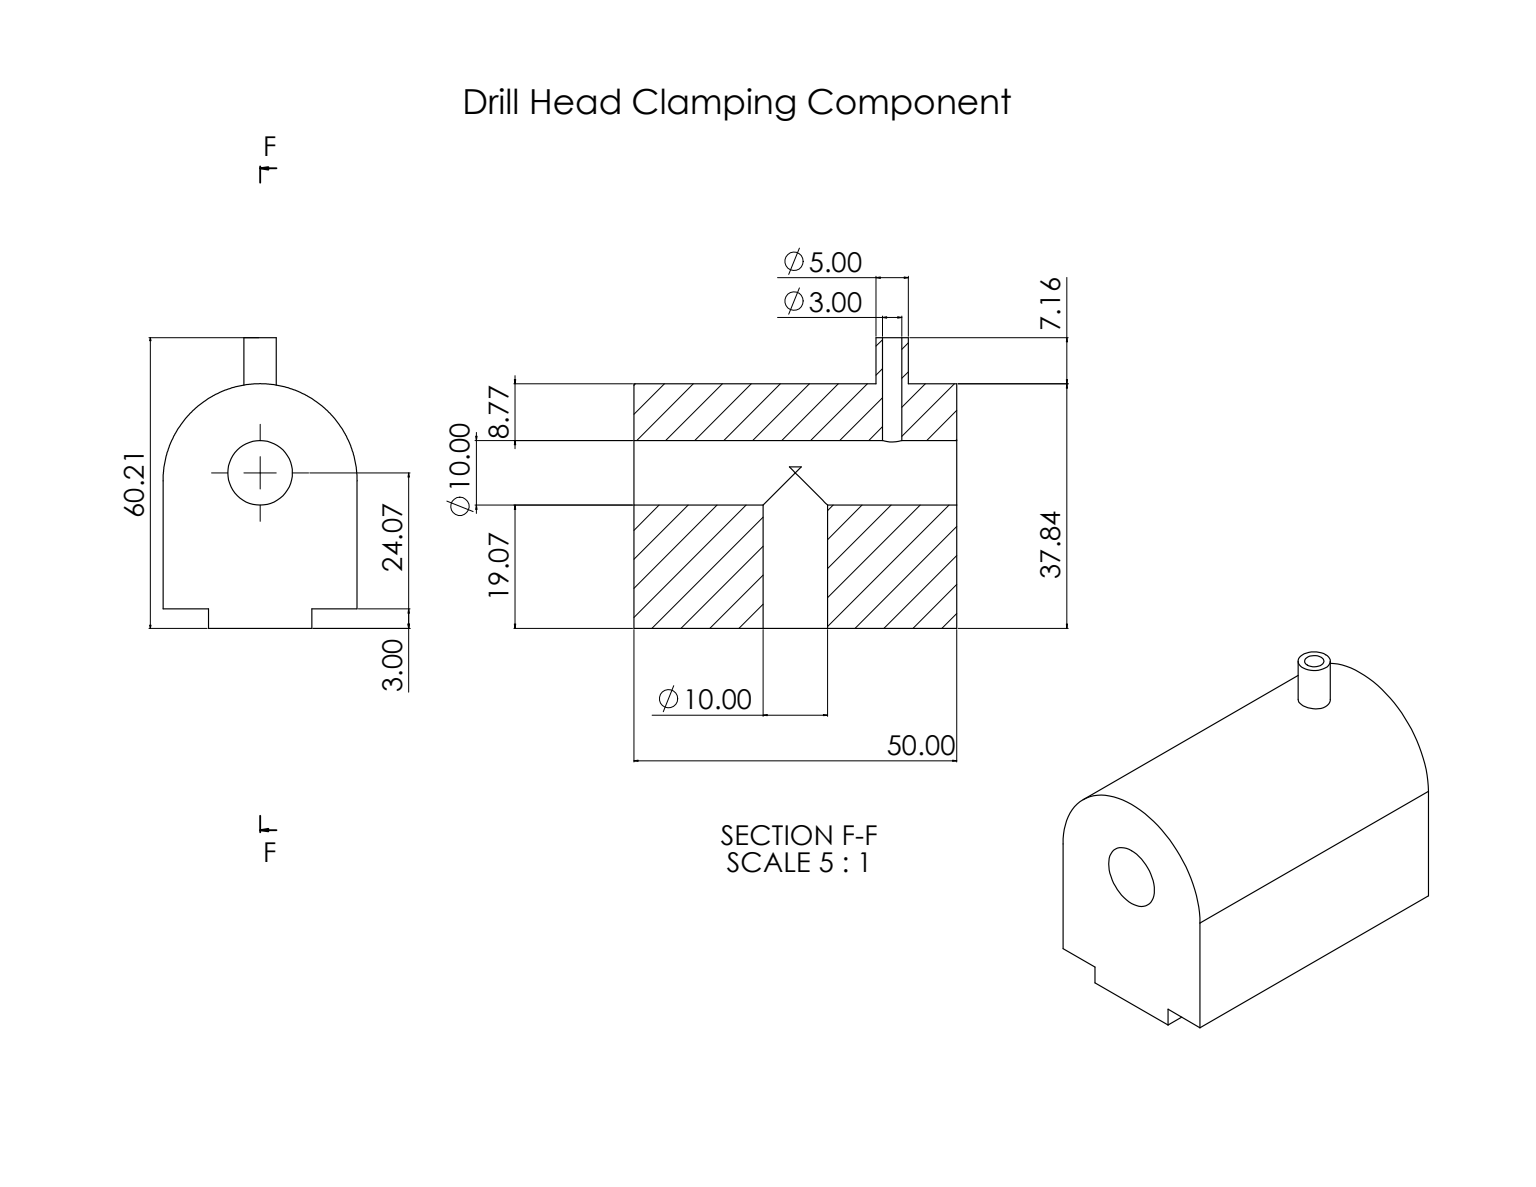
ISO-10303-21;
HEADER;
FILE_DESCRIPTION (('STEP AP214'),
    '1' );
FILE_NAME ('Drill Head Clamping Component.step',
    '2026-10-26T22:46:44',
    ( '' ),
    ( '' ),
    'SwSTEP 2.0',
    'SolidWorks 2025',
    '' );
FILE_SCHEMA (( 'AUTOMOTIVE_DESIGN' ));
ENDSEC;

DATA;
#26=DIRECTION ( 'NONE',  ( 0.5000000000000044409, -0.8660254037844360431, -4.006172263299080068E-16 ) ) ;
#120=CARTESIAN_POINT ( 'NONE',  ( 184.9952905943350743, 3.535126980567765642, 0.9999999999999187317 ) ) ;
#154=CARTESIAN_POINT ( 'NONE',  ( 189.6713070174558311, 31.72030020615783030, -9.000000000000065725 ) ) ;
#219=CARTESIAN_POINT ( 'NONE',  ( 203.2433706042751282, 14.07066088650062241, -14.00000000000004974 ) ) ;
#263=EDGE_CURVE ( 'NONE', #15664, #11736, #7688, .T. ) ;
#270=VERTEX_POINT ( 'NONE', #17044 ) ;
#297=AXIS2_PLACEMENT_3D ( 'NONE', #15625, #6046, #20370 ) ;
#298=CARTESIAN_POINT ( 'NONE',  ( 191.0833833835251880, 36.99024094849657018, -18.91295074164679235 ) ) ;
#299=( BOUNDED_CURVE ( )  B_SPLINE_CURVE ( 3, ( #3480, #412, #16318, #298 ),
 .UNSPECIFIED., .F., .F. ) 
 B_SPLINE_CURVE_WITH_KNOTS ( ( 4, 4 ),
 ( 1.570796326794896114, 1.757668500643543075 ),
 .UNSPECIFIED. ) 
 CURVE ( )  GEOMETRIC_REPRESENTATION_ITEM ( )  RATIONAL_B_SPLINE_CURVE ( ( 1.000000000000000000, 0.9970920157757051649, 0.9970920157757051649, 1.000000000000000000 ) ) 
 REPRESENTATION_ITEM ( '' )  );
#319=EDGE_CURVE ( 'NONE', #17948, #11709, #17482, .T. ) ;
#339=CARTESIAN_POINT ( 'NONE',  ( 203.2094460813901833, 24.04198982742622448, -13.33402418452071814 ) ) ;
#363=VECTOR ( 'NONE', #26, 1000.000000000000114 ) ;
#394=ORIENTED_EDGE ( 'NONE', *, *, #20392, .T. ) ;
#410=ORIENTED_EDGE ( 'NONE', *, *, #16561, .T. ) ;
#412=CARTESIAN_POINT ( 'NONE',  ( 190.8575367324608294, 36.14736977200441004, -19.00000000000003908 ) ) ;
#450=CARTESIAN_POINT ( 'NONE',  ( 201.8234976231972553, 26.52995303002162331, -14.00000000000004619 ) ) ;
#462=LINE ( 'NONE', #18261, #4286 ) ;
#465=ORIENTED_EDGE ( 'NONE', *, *, #17085, .T. ) ;
#502=ORIENTED_EDGE ( 'NONE', *, *, #9754, .F. ) ;
#521=CARTESIAN_POINT ( 'NONE',  ( 190.7433706042750146, 35.72129598111152404, -19.00000000000003908 ) ) ;
#586=CARTESIAN_POINT ( 'NONE',  ( 191.5478494775925640, 36.18576207517880050, -14.00000000000006395 ) ) ;
#601=ORIENTED_EDGE ( 'NONE', *, *, #10960, .T. ) ;
#656=ORIENTED_EDGE ( 'NONE', *, *, #14023, .F. ) ;
#665=EDGE_CURVE ( 'NONE', #15359, #17948, #14273, .T. ) ;
#674=FACE_OUTER_BOUND ( 'NONE', #15043, .T. ) ;
#709=VECTOR ( 'NONE', #16147, 1000.000000000000000 ) ;
#716=DIRECTION ( 'NONE',  ( 0.5000000000000046629, -0.8660254037844360431, -4.006172263299081054E-16 ) ) ;
#719=ADVANCED_FACE ( 'NONE', ( #9867 ), #20902, .F. ) ;
#723=EDGE_CURVE ( 'NONE', #3430, #270, #9321, .T. ) ;
#750=LINE ( 'NONE', #16854, #10405 ) ;
#778=ORIENTED_EDGE ( 'NONE', *, *, #1234, .T. ) ;
#783=PRODUCT ( 'Drill Head Clamping Component', 'Drill Head Clamping Component', '', ( #7533 ) ) ;
#784=VERTEX_POINT ( 'NONE', #1941 ) ;
#837=CARTESIAN_POINT ( 'NONE',  ( 201.9048419744482317, 26.22127161638350756, -13.08418984338544355 ) ) ;
#849=LINE ( 'NONE', #4134, #8722 ) ;
#861=EDGE_CURVE ( 'NONE', #17088, #19623, #11689, .T. ) ;
#939=CARTESIAN_POINT ( 'NONE',  ( 201.8234976231972269, 26.52995303002161620, -13.90027237864162757 ) ) ;
#942=VECTOR ( 'NONE', #9777, 1000.000000000000114 ) ;
#946=ORIENTED_EDGE ( 'NONE', *, *, #6874, .T. ) ;
#962=EDGE_CURVE ( 'NONE', #14228, #10601, #3174, .T. ) ;
#978=ORIENTED_EDGE ( 'NONE', *, *, #6131, .F. ) ;
#1019=DIRECTION ( 'NONE',  ( -3.517351572405780687E-16, 2.595185392108431646E-16, -1.000000000000000000 ) ) ;
#1071=DIRECTION ( 'NONE',  ( -0.8660254037844361541, -0.5000000000000045519, -4.336808689942050770E-16 ) ) ;
#1074=PLANE ( 'NONE',  #8585 ) ;
#1129=EDGE_CURVE ( 'NONE', #19322, #784, #1828, .T. ) ;
#1234=EDGE_CURVE ( 'NONE', #10655, #15958, #18417, .T. ) ;
#1236=ORIENTED_EDGE ( 'NONE', *, *, #11597, .T. ) ;
#1267=EDGE_CURVE ( 'NONE', #13023, #3226, #5866, .T. ) ;
#1274=DIRECTION ( 'NONE',  ( 0.000000000000000000, 0.000000000000000000, 1.000000000000000000 ) ) ;
#1300=CARTESIAN_POINT ( 'NONE',  ( 210.6607590550263183, 28.44678604684768786, -16.18447207777755281 ) ) ;
#1305=DIRECTION ( 'NONE',  ( 0.5000000000000044409, -0.8660254037844360431, 0.000000000000000000 ) ) ;
#1311=DIRECTION ( 'NONE',  ( 0.5000000000000046629, -0.8660254037844360431, -4.006172263299081054E-16 ) ) ;
#1339=CARTESIAN_POINT ( 'NONE',  ( 203.3234976231972553, 23.93187681866832861, -14.00000000000004441 ) ) ;
#1341=DIRECTION ( 'NONE',  ( 0.8660254037844360431, 0.5000000000000044409, 4.336808689942049290E-16 ) ) ;
#1403=CARTESIAN_POINT ( 'NONE',  ( 215.1694833127197057, 20.95620526910698445, -14.00000000000008527 ) ) ;
#1430=VECTOR ( 'NONE', #5416, 1000.000000000000227 ) ;
#1434=CARTESIAN_POINT ( 'NONE',  ( 188.9132435853528591, 28.89116896218934016, -16.92893218813457068 ) ) ;
#1459=DIRECTION ( 'NONE',  ( 0.5000000000000044409, -0.8660254037844360431, -4.006172263299080068E-16 ) ) ;
#1464=DIRECTION ( 'NONE',  ( 0.5000000000000057732, -0.8660254037844353769, 0.000000000000000000 ) ) ;
#1500=DIRECTION ( 'NONE',  ( -0.5000000000000025535, 0.8660254037844372643, 0.000000000000000000 ) ) ;
#1504=CARTESIAN_POINT ( 'NONE',  ( 210.0699630922315748, 29.36925333534437499, -16.49993777872327527 ) ) ;
#1510=PLANE ( 'NONE',  #13226 ) ;
#1512=DIRECTION ( 'NONE',  ( -0.8660254037844361541, -0.5000000000000045519, 8.850264995343375625E-15 ) ) ;
#1579=CIRCLE ( 'NONE', #13424, 15.00000000000001954 ) ;
#1607=CARTESIAN_POINT ( 'NONE',  ( 209.1488401613018198, 31.20282942076142518, -15.65137675853565646 ) ) ;
#1621=DIRECTION ( 'NONE',  ( 0.8660254037844361541, 0.5000000000000044409, 0.000000000000000000 ) ) ;
#1642=CARTESIAN_POINT ( 'NONE',  ( 188.9132435853528591, 28.89116896218934016, -11.07106781186553768 ) ) ;
#1649=CARTESIAN_POINT ( 'NONE',  ( 210.8166463470705310, 28.23117696587115333, -12.01093917984183790 ) ) ;
#1691=CARTESIAN_POINT ( 'NONE',  ( 184.9952905943350743, 3.535126980567779409, -29.00000000000008882 ) ) ;
#1702=ORIENTED_EDGE ( 'NONE', *, *, #12220, .F. ) ;
#1749=ADVANCED_FACE ( 'NONE', ( #8633 ), #15030, .F. ) ;
#1752=CARTESIAN_POINT ( 'NONE',  ( 211.3365836822136430, 27.55273924158569798, -13.19013634410915969 ) ) ;
#1828=CIRCLE ( 'NONE', #18066, 1.499999999999993783 ) ;
#1869=( NAMED_UNIT ( * ) PLANE_ANGLE_UNIT ( ) SI_UNIT ( $, .RADIAN. ) );
#1875=AXIS2_PLACEMENT_3D ( 'NONE', #4980, #8260, #18132 ) ;
#1896=ADVANCED_FACE ( 'NONE', ( #19128 ), #2497, .F. ) ;
#1902=DIRECTION ( 'NONE',  ( -2.003086131649568876E-16, 3.469446951953589044E-16, -1.000000000000000000 ) ) ;
#1934=CARTESIAN_POINT ( 'NONE',  ( 201.8352585209308359, 26.48094985263767498, -13.60979871437957911 ) ) ;
#1941=CARTESIAN_POINT ( 'NONE',  ( 217.1183575532814416, 31.89634291273570810, -14.00000000000004441 ) ) ;
#1972=CARTESIAN_POINT ( 'NONE',  ( 203.2093925786781767, 24.04204282662517400, -14.66612357830583946 ) ) ;
#1979=EDGE_LOOP ( 'NONE', ( #13601, #10740, #15513, #394 ) ) ;
#1980=ORIENTED_EDGE ( 'NONE', *, *, #665, .T. ) ;
#1988=ORIENTED_EDGE ( 'NONE', *, *, #20436, .F. ) ;
#1996=ORIENTED_EDGE ( 'NONE', *, *, #12220, .T. ) ;
#2021=ORIENTED_EDGE ( 'NONE', *, *, #14700, .T. ) ;
#2053=LINE ( 'NONE', #5528, #1430 ) ;
#2091=EDGE_LOOP ( 'NONE', ( #13331, #5335, #14741, #12606, #6343, #16377, #14233, #11644, #18125 ) ) ;
#2162=CARTESIAN_POINT ( 'NONE',  ( 202.1791022559531541, 13.45620526910691694, -14.00000000000008527 ) ) ;
#2272=EDGE_LOOP ( 'NONE', ( #3905, #20020, #978 ) ) ;
#2294=DIRECTION ( 'NONE',  ( -0.5000000000000034417, 0.8660254037844364872, 0.000000000000000000 ) ) ;
#2335=ORIENTED_EDGE ( 'NONE', *, *, #4367, .F. ) ;
#2396=DIRECTION ( 'NONE',  ( -0.8660254037844360431, -0.5000000000000045519, -4.336808689942049784E-16 ) ) ;
#2409=CARTESIAN_POINT ( 'NONE',  ( 173.9132435853527454, 54.87193107572242212, -14.00000000000002842 ) ) ;
#2410=CIRCLE ( 'NONE', #14943, 4.999999999999978684 ) ;
#2415=ORIENTED_EDGE ( 'NONE', *, *, #11750, .F. ) ;
#2433=ORIENTED_EDGE ( 'NONE', *, *, #20050, .T. ) ;
#2462=ORIENTED_EDGE ( 'NONE', *, *, #1234, .F. ) ;
#2476=( BOUNDED_CURVE ( )  B_SPLINE_CURVE ( 3, ( #8745, #4299, #15659, #5761 ),
 .UNSPECIFIED., .F., .F. ) 
 B_SPLINE_CURVE_WITH_KNOTS ( ( 4, 4 ),
 ( 1.383924152946250041, 1.570796326794896558 ),
 .UNSPECIFIED. ) 
 CURVE ( )  GEOMETRIC_REPRESENTATION_ITEM ( )  RATIONAL_B_SPLINE_CURVE ( ( 1.000000000000000000, 0.9970920157757051649, 0.9970920157757051649, 1.000000000000000000 ) ) 
 REPRESENTATION_ITEM ( '' )  );
#2482=ORIENTED_EDGE ( 'NONE', *, *, #20787, .T. ) ;
#2485=LINE ( 'NONE', #7338, #20363 ) ;
#2497=CYLINDRICAL_SURFACE ( 'NONE', #8268, 4.999999999999975131 ) ;
#2514=CARTESIAN_POINT ( 'NONE',  ( 177.1791022559528983, 56.75747545832873442, -29.00000000000007105 ) ) ;
#2536=CARTESIAN_POINT ( 'NONE',  ( 201.8258408404966531, 26.51993709131365762, -13.80232238285611857 ) ) ;
#2568=CIRCLE ( 'NONE', #1875, 15.00000000000001954 ) ;
#2571=AXIS2_PLACEMENT_3D ( 'NONE', #13843, #5653, #14253 ) ;
#2577=EDGE_LOOP ( 'NONE', ( #4212, #6761 ) ) ;
#2578=CARTESIAN_POINT ( 'NONE',  ( 203.2433706042751282, 14.07066088650062241, -14.00000000000004974 ) ) ;
#2611=ORIENTED_EDGE ( 'NONE', *, *, #17969, .F. ) ;
#2632=CARTESIAN_POINT ( 'NONE',  ( 216.3683575532813848, 33.19538101841231992, -14.00000000000004441 ) ) ;
#2635=CARTESIAN_POINT ( 'NONE',  ( 207.5734976231972837, 16.57066088650062241, -14.00000000000004974 ) ) ;
#2657=PRODUCT_DEFINITION_SHAPE ( 'NONE', 'NONE',  #13142 ) ;
#2676=( GEOMETRIC_REPRESENTATION_CONTEXT ( 3 ) GLOBAL_UNCERTAINTY_ASSIGNED_CONTEXT ( ( #17640 ) ) GLOBAL_UNIT_ASSIGNED_CONTEXT ( ( #13415, #7036, #20186 ) ) REPRESENTATION_CONTEXT ( 'NONE', 'WORKASPACE' ) );
#2716=FACE_OUTER_BOUND ( 'NONE', #2577, .T. ) ;
#2720=VERTEX_POINT ( 'NONE', #6853 ) ;
#2721=ORIENTED_EDGE ( 'NONE', *, *, #14023, .T. ) ;
#2733=DIRECTION ( 'NONE',  ( 0.5000000000000015543, -0.8660254037844377084, 0.000000000000000000 ) ) ;
#2811=VECTOR ( 'NONE', #20786, 1000.000000000000114 ) ;
#2817=LINE ( 'NONE', #17224, #20375 ) ;
#2860=VERTEX_POINT ( 'NONE', #10871 ) ;
#2888=CARTESIAN_POINT ( 'NONE',  ( 209.4688803963327928, 30.49173192974595992, -16.24689738482229728 ) ) ;
#2890=EDGE_LOOP ( 'NONE', ( #656, #6702, #11561, #1980, #5146 ) ) ;
#2893=DIRECTION ( 'NONE',  ( 0.5000000000000044409, -0.8660254037844360431, 0.000000000000000000 ) ) ;
#2924=VECTOR ( 'NONE', #8682, 1000.000000000000114 ) ;
#2937=ORIENTED_EDGE ( 'NONE', *, *, #263, .T. ) ;
#3047=DIRECTION ( 'NONE',  ( 0.5000000000000046629, -0.8660254037844360431, -4.006172263299081054E-16 ) ) ;
#3097=CARTESIAN_POINT ( 'NONE',  ( 208.9194833127196489, 31.78152281641241572, -14.16331216883973987 ) ) ;
#3104=CARTESIAN_POINT ( 'NONE',  ( 190.7433706042750146, 35.72129598111152404, -9.000000000000062172 ) ) ;
#3137=CARTESIAN_POINT ( 'NONE',  ( 209.4677058171011197, 30.49417139021348078, -11.75443427544081310 ) ) ;
#3174=CIRCLE ( 'NONE', #10608, 5.000000000000002665 ) ;
#3193=CARTESIAN_POINT ( 'NONE',  ( 210.4099586451761184, 28.82287685411301936, -16.37159109994057360 ) ) ;
#3219=VECTOR ( 'NONE', #13608, 1000.000000000000114 ) ;
#3226=VERTEX_POINT ( 'NONE', #18596 ) ;
#3251=DIRECTION ( 'NONE',  ( -0.8660254037844360431, -0.5000000000000045519, -4.336808689942050277E-16 ) ) ;
#3295=CARTESIAN_POINT ( 'NONE',  ( 209.8259871216629335, 29.79736469536937093, -16.48372795108025812 ) ) ;
#3338=CARTESIAN_POINT ( 'NONE',  ( 209.6745996013020772, 30.08081452043873227, -11.58037181831264029 ) ) ;
#3358=B_SPLINE_CURVE_WITH_KNOTS ( 'NONE', 3,
 ( #14921, #7255, #8744, #1972, #15242, #19978, #13638, #20091, #16912, #15037, #8536, #12042, #18607, #18289, #13738, #10320, #15139, #11829, #16595, #8639, #5441, #3763, #11940, #18509, #5235, #5552, #13425, #15350 ),
 .UNSPECIFIED., .F., .F.,
 ( 4, 2, 2, 2, 2, 2, 2, 2, 2, 2, 2, 2, 2, 4 ),
 ( 0.004717002832140601738, 0.005306469451344702354, 0.005601202760946753095, 0.005895936070548802969, 0.006485402689752946953, 0.006780135999355018511, 0.007074869308957089202, 0.007369602618559159893, 0.007664335928161231451, 0.008253802547365364159, 0.008548535856967442656, 0.008843269166569519418, 0.009138002476171597915, 0.009432735785773674678 ),
 .UNSPECIFIED. ) ;
#3368=AXIS2_PLACEMENT_3D ( 'NONE', #10550, #17528, #1621 ) ;
#3392=CIRCLE ( 'NONE', #13898, 2.499999999999994671 ) ;
#3430=VERTEX_POINT ( 'NONE', #15661 ) ;
#3480=CARTESIAN_POINT ( 'NONE',  ( 190.7433706042750146, 35.72129598111152404, -19.00000000000003908 ) ) ;
#3710=DIRECTION ( 'NONE',  ( 0.5000000000000044409, -0.8660254037844360431, -4.006172263299080068E-16 ) ) ;
#3734=CARTESIAN_POINT ( 'NONE',  ( 159.9952905943348469, 46.83639716978957068, 0.9999999999999386047 ) ) ;
#3754=SHAPE_REPRESENTATION_RELATIONSHIP ( 'NONE' , 'NONE' ,  #9638, #5517 ) ;
#3756=VERTEX_POINT ( 'NONE', #15220 ) ;
#3762=ORIENTED_EDGE ( 'NONE', *, *, #16561, .F. ) ;
#3763=CARTESIAN_POINT ( 'NONE',  ( 201.8742535751798073, 26.32928792145338548, -14.75325243452065749 ) ) ;
#3767=DIRECTION ( 'NONE',  ( 0.8660254037844360431, 0.5000000000000045519, 4.336808689942049784E-16 ) ) ;
#3773=ORIENTED_EDGE ( 'NONE', *, *, #14700, .F. ) ;
#3778=ORIENTED_EDGE ( 'NONE', *, *, #319, .F. ) ;
#3805=ORIENTED_EDGE ( 'NONE', *, *, #13350, .T. ) ;
#3828=DIRECTION ( 'NONE',  ( 0.8660254037844360431, 0.5000000000000045519, 4.336808689942050277E-16 ) ) ;
#3905=ORIENTED_EDGE ( 'NONE', *, *, #8879, .F. ) ;
#3927=LINE ( 'NONE', #8806, #11231 ) ;
#3983=DIRECTION ( 'NONE',  ( -0.8660254037844360431, -0.5000000000000044409, -4.336808689942049290E-16 ) ) ;
#4002=LINE ( 'NONE', #18212, #14326 ) ;
#4009=CARTESIAN_POINT ( 'NONE',  ( 202.1874421558074744, 25.46507160306319406, -12.54005369788149693 ) ) ;
#4012=VERTEX_POINT ( 'NONE', #18044 ) ;
#4100=AXIS2_PLACEMENT_3D ( 'NONE', #17999, #3251, #1464 ) ;
#4134=CARTESIAN_POINT ( 'NONE',  ( 159.9952905943348469, 46.83639716978957068, 0.9999999999999386047 ) ) ;
#4180=FACE_OUTER_BOUND ( 'NONE', #1979, .T. ) ;
#4198=ADVANCED_FACE ( 'NONE', ( #5801, #12295 ), #7500, .T. ) ;
#4207=( BOUNDED_CURVE ( )  B_SPLINE_CURVE ( 3, ( #16447, #11575, #14992, #18045 ),
 .UNSPECIFIED., .F., .F. ) 
 B_SPLINE_CURVE_WITH_KNOTS ( ( 4, 4 ),
 ( 4.525516806536070469, 4.712388980384689674 ),
 .UNSPECIFIED. ) 
 CURVE ( )  GEOMETRIC_REPRESENTATION_ITEM ( )  RATIONAL_B_SPLINE_CURVE ( ( 1.000000000000000000, 0.9970920157757060531, 0.9970920157757060531, 1.000000000000000000 ) ) 
 REPRESENTATION_ITEM ( '' )  );
#4212=ORIENTED_EDGE ( 'NONE', *, *, #10396, .T. ) ;
#4227=VERTEX_POINT ( 'NONE', #7385 ) ;
#4286=VECTOR ( 'NONE', #18474, 1000.000000000000114 ) ;
#4299=CARTESIAN_POINT ( 'NONE',  ( 191.5936596622673278, 35.49346171468947375, -18.97089895516968028 ) ) ;
#4323=CARTESIAN_POINT ( 'NONE',  ( 191.0833833835251880, 36.99024094849657018, -18.91295074164679235 ) ) ;
#4340=EDGE_LOOP ( 'NONE', ( #11227, #4467, #18364, #14808, #8937, #2021, #8246, #17322, #3805 ) ) ;
#4367=EDGE_CURVE ( 'NONE', #11709, #17948, #17634, .T. ) ;
#4383=CARTESIAN_POINT ( 'NONE',  ( 159.9952905943347901, 46.83639716978955647, -22.00000000000007816 ) ) ;
#4388=DIRECTION ( 'NONE',  ( 1.561274065702232331E-18, -4.616915249250367527E-16, 1.000000000000000000 ) ) ;
#4461=DIRECTION ( 'NONE',  ( -0.5000000000000045519, 0.8660254037844360431, 4.006172263299081054E-16 ) ) ;
#4467=ORIENTED_EDGE ( 'NONE', *, *, #16106, .T. ) ;
#4485=LINE ( 'NONE', #12339, #5183 ) ;
#4486=FACE_OUTER_BOUND ( 'NONE', #4840, .T. ) ;
#4584=CARTESIAN_POINT ( 'NONE',  ( 217.6183575532813848, 31.03031750895123508, -14.00000000000004441 ) ) ;
#4598=CARTESIAN_POINT ( 'NONE',  ( 191.5478494775925640, 36.18576207517880050, -14.00000000000006395 ) ) ;
#4622=EDGE_CURVE ( 'NONE', #9607, #13077, #8793, .T. ) ;
#4652=DIRECTION ( 'NONE',  ( -0.8660254037844344888, -0.5000000000000069944, 0.000000000000000000 ) ) ;
#4715=EDGE_CURVE ( 'NONE', #18333, #14531, #8447, .T. ) ;
#4717=CARTESIAN_POINT ( 'NONE',  ( 209.1489059746362216, 31.20269758479947697, -12.34862215763092763 ) ) ;
#4731=ADVANCED_FACE ( 'NONE', ( #11058 ), #7759, .T. ) ;
#4777=CARTESIAN_POINT ( 'NONE',  ( 216.3683575532814416, 33.19538101841234834, -14.00000000000004441 ) ) ;
#4831=VECTOR ( 'NONE', #15686, 1000.000000000000114 ) ;
#4840=EDGE_LOOP ( 'NONE', ( #9568, #10904, #6846, #9175 ) ) ;
#4867=ORIENTED_EDGE ( 'NONE', *, *, #7845, .T. ) ;
#4884=ORIENTED_EDGE ( 'NONE', *, *, #6131, .T. ) ;
#4886=CARTESIAN_POINT ( 'NONE',  ( 210.1535261002520087, 29.22995462719417148, -16.48401562083277483 ) ) ;
#4894=EDGE_LOOP ( 'NONE', ( #11762, #6045, #20022 ) ) ;
#4922=CARTESIAN_POINT ( 'NONE',  ( 159.9952905943347901, 46.83639716978955647, -22.00000000000007816 ) ) ;
#4957=CARTESIAN_POINT ( 'NONE',  ( 157.3972143829815309, 45.33639716978957068, -22.00000000000007816 ) ) ;
#4973=ORIENTED_EDGE ( 'NONE', *, *, #6796, .F. ) ;
#4980=CARTESIAN_POINT ( 'NONE',  ( 177.1791022559528983, 56.75747545832872731, -14.00000000000006395 ) ) ;
#5014=EDGE_CURVE ( 'NONE', #784, #19322, #12224, .T. ) ;
#5022=DIRECTION ( 'NONE',  ( -0.8660254037844361541, -0.5000000000000045519, -8.850264995343378780E-15 ) ) ;
#5033=( NAMED_UNIT ( * ) SI_UNIT ( $, .STERADIAN. ) SOLID_ANGLE_UNIT ( ) );
#5076=DIRECTION ( 'NONE',  ( 0.5000000000000046629, -0.8660254037844360431, -4.006172263299081054E-16 ) ) ;
#5083=CARTESIAN_POINT ( 'NONE',  ( 191.5478494775925640, 36.18576207517880050, -14.00000000000006395 ) ) ;
#5118=CARTESIAN_POINT ( 'NONE',  ( 188.9132435853528591, 28.89116896218935082, -14.00000000000004086 ) ) ;
#5138=CARTESIAN_POINT ( 'NONE',  ( 159.9952905943347901, 46.83639716978954226, -6.000000000000052403 ) ) ;
#5146=ORIENTED_EDGE ( 'NONE', *, *, #319, .T. ) ;
#5170=ORIENTED_EDGE ( 'NONE', *, *, #7845, .F. ) ;
#5183=VECTOR ( 'NONE', #14256, 1000.000000000000114 ) ;
#5193=CARTESIAN_POINT ( 'NONE',  ( 202.2752485137783083, 25.28694651298519958, -12.50009056643368943 ) ) ;
#5235=CARTESIAN_POINT ( 'NONE',  ( 201.8352900073124658, 26.48082042610822029, -14.39073202032135335 ) ) ;
#5240=CARTESIAN_POINT ( 'NONE',  ( 216.3683575532813848, 33.19538101841231992, -14.00000000000004441 ) ) ;
#5284=CARTESIAN_POINT ( 'NONE',  ( 184.9952905943350459, 3.535126980567751431, -22.00000000000009948 ) ) ;
#5285=AXIS2_PLACEMENT_3D ( 'NONE', #4922, #5022, #11398 ) ;
#5294=CARTESIAN_POINT ( 'NONE',  ( 201.9876756982950781, 25.95812089196162020, -12.80147382135962353 ) ) ;
#5295=EDGE_CURVE ( 'NONE', #17359, #17685, #10465, .T. ) ;
#5335=ORIENTED_EDGE ( 'NONE', *, *, #15580, .F. ) ;
#5341=DIRECTION ( 'NONE',  ( 0.5000000000000015543, -0.8660254037844377084, 0.000000000000000000 ) ) ;
#5395=AXIS2_PLACEMENT_3D ( 'NONE', #16816, #3767, #2294 ) ;
#5416=DIRECTION ( 'NONE',  ( 0.8660254037844344888, 0.5000000000000069944, 0.000000000000000000 ) ) ;
#5426=ORIENTED_EDGE ( 'NONE', *, *, #14613, .F. ) ;
#5441=CARTESIAN_POINT ( 'NONE',  ( 201.9048576179487213, 26.22121821873378877, -14.91588034066295521 ) ) ;
#5443=FACE_BOUND ( 'NONE', #20780, .T. ) ;
#5462=AXIS2_PLACEMENT_3D ( 'NONE', #2162, #8615, #7123 ) ;
#5517=ADVANCED_BREP_SHAPE_REPRESENTATION ( '', ( #10635, #18233 ), #2676 ) ;
#5528=CARTESIAN_POINT ( 'NONE',  ( 182.3972143829817867, 2.035126980567763866, -22.00000000000009948 ) ) ;
#5552=CARTESIAN_POINT ( 'NONE',  ( 201.8258405466010572, 26.51993739047028242, -14.19778417152125805 ) ) ;
#5569=ORIENTED_EDGE ( 'NONE', *, *, #17776, .T. ) ;
#5653=DIRECTION ( 'NONE',  ( 0.8660254037844360431, 0.5000000000000045519, 4.336808689942049784E-16 ) ) ;
#5708=CARTESIAN_POINT ( 'NONE',  ( 177.1791022559528983, 56.75747545832872731, -29.00000000000007105 ) ) ;
#5715=DIRECTION ( 'NONE',  ( -0.5000000000000025535, 0.8660254037844372643, 0.000000000000000000 ) ) ;
#5761=CARTESIAN_POINT ( 'NONE',  ( 190.7433706042750146, 35.72129598111152404, -19.00000000000003908 ) ) ;
#5781=DIRECTION ( 'NONE',  ( -0.8660254037844361541, -0.5000000000000044409, 0.000000000000000000 ) ) ;
#5798=ORIENTED_EDGE ( 'NONE', *, *, #6374, .F. ) ;
#5799=CARTESIAN_POINT ( 'NONE',  ( 203.0531299009467148, 24.20278031722661183, -13.00893198973463960 ) ) ;
#5801=FACE_BOUND ( 'NONE', #8961, .T. ) ;
#5807=CARTESIAN_POINT ( 'NONE',  ( 159.9952905943348469, 46.83639716978957068, 0.9999999999999386047 ) ) ;
#5854=EDGE_LOOP ( 'NONE', ( #11800, #2721, #15594, #20249, #2415 ) ) ;
#5866=CIRCLE ( 'NONE', #14025, 4.999999999999976907 ) ;
#5886=EDGE_CURVE ( 'NONE', #14632, #18333, #14649, .T. ) ;
#5920=CARTESIAN_POINT ( 'NONE',  ( 191.5478494775925640, 36.18576207517880050, -14.00000000000006395 ) ) ;
#5924=DIRECTION ( 'NONE',  ( -0.5000000000000045519, 0.8660254037844360431, 4.006172263299081054E-16 ) ) ;
#5927=CLOSED_SHELL ( 'NONE', ( #12509, #8115, #8098, #1896, #8560, #6051, #11221, #4731, #14582, #16267, #7579, #4198, #13178, #13707, #13696, #17936, #19015, #13259, #19429, #12566, #1749, #6884, #18238, #719 ) ) ;
#6045=ORIENTED_EDGE ( 'NONE', *, *, #18884, .F. ) ;
#6046=DIRECTION ( 'NONE',  ( -0.8660254037844360431, -0.5000000000000045519, -4.336808689942049784E-16 ) ) ;
#6051=ADVANCED_FACE ( 'NONE', ( #4486 ), #19009, .T. ) ;
#6054=CARTESIAN_POINT ( 'NONE',  ( 191.5936596622672141, 35.49346171468950928, -9.029101044830413869 ) ) ;
#6070=CARTESIAN_POINT ( 'NONE',  ( 178.2433706042749009, 57.37193107572242923, -14.00000000000002842 ) ) ;
#6129=AXIS2_PLACEMENT_3D ( 'NONE', #10628, #4388, #17323 ) ;
#6131=EDGE_CURVE ( 'NONE', #3430, #2720, #15854, .T. ) ;
#6142=ORIENTED_EDGE ( 'NONE', *, *, #9754, .T. ) ;
#6155=CARTESIAN_POINT ( 'NONE',  ( 209.2927537897656407, 30.87096182040829007, -15.98783141827518328 ) ) ;
#6178=AXIS2_PLACEMENT_3D ( 'NONE', #5083, #11567, #8904 ) ;
#6195=ORIENTED_EDGE ( 'NONE', *, *, #1267, .T. ) ;
#6297=CARTESIAN_POINT ( 'NONE',  ( 209.0110543411082062, 31.54257417018269649, -12.89263383701904608 ) ) ;
#6343=ORIENTED_EDGE ( 'NONE', *, *, #9238, .F. ) ;
#6356=CARTESIAN_POINT ( 'NONE',  ( 209.6034591737553683, 30.21950843401080533, -16.37243376991346011 ) ) ;
#6374=EDGE_CURVE ( 'NONE', #9882, #2860, #3927, .T. ) ;
#6375=CARTESIAN_POINT ( 'NONE',  ( 186.7423748293213066, 36.79335956793067197, -9.000000000000063949 ) ) ;
#6389=DIRECTION ( 'NONE',  ( 0.5000000000000015543, -0.8660254037844377084, 0.000000000000000000 ) ) ;
#6455=CARTESIAN_POINT ( 'NONE',  ( 211.4194833127196489, 27.45139579749023540, -14.00000000000004974 ) ) ;
#6499=EDGE_LOOP ( 'NONE', ( #14458, #410, #15745, #19321, #8326, #17712, #17113, #4867, #5569, #20005, #9614, #7570 ) ) ;
#6541=ORIENTED_EDGE ( 'NONE', *, *, #16106, .F. ) ;
#6553=CARTESIAN_POINT ( 'NONE',  ( 173.9132435853527454, 54.87193107572242212, -14.00000000000002842 ) ) ;
#6592=ORIENTED_EDGE ( 'NONE', *, *, #8222, .T. ) ;
#6601=CARTESIAN_POINT ( 'NONE',  ( 211.1008594470266360, 27.84852471586090772, -12.46092303668267398 ) ) ;
#6606=DIRECTION ( 'NONE',  ( 0.5000000000000057732, -0.8660254037844353769, 0.000000000000000000 ) ) ;
#6666=FACE_OUTER_BOUND ( 'NONE', #5854, .T. ) ;
#6702=ORIENTED_EDGE ( 'NONE', *, *, #723, .F. ) ;
#6705=CARTESIAN_POINT ( 'NONE',  ( 211.4194833127196205, 27.45139579749023540, -13.83454964029852086 ) ) ;
#6708=CARTESIAN_POINT ( 'NONE',  ( 169.8972143829816730, 23.68576207517868326, -14.00000000000007461 ) ) ;
#6739=DIRECTION ( 'NONE',  ( 0.5000000000000044409, -0.8660254037844360431, -4.006172263299080068E-16 ) ) ;
#6742=AXIS2_PLACEMENT_3D ( 'NONE', #5240, #2396, #5341 ) ;
#6761=ORIENTED_EDGE ( 'NONE', *, *, #962, .T. ) ;
#6770=DIRECTION ( 'NONE',  ( 7.930164461608273850E-15, 3.965082230804136925E-15, -1.000000000000000000 ) ) ;
#6796=EDGE_CURVE ( 'NONE', #10831, #7353, #3358, .T. ) ;
#6816=CYLINDRICAL_SURFACE ( 'NONE', #15604, 15.00000000000001954 ) ;
#6837=ORIENTED_EDGE ( 'NONE', *, *, #15027, .F. ) ;
#6846=ORIENTED_EDGE ( 'NONE', *, *, #20883, .T. ) ;
#6853=CARTESIAN_POINT ( 'NONE',  ( 192.0123155716598262, 35.38128320186126530, -9.087049258353282255 ) ) ;
#6874=EDGE_CURVE ( 'NONE', #9882, #3756, #12856, .T. ) ;
#6875=CARTESIAN_POINT ( 'NONE',  ( 183.9132435853528023, 37.55142300003368661, -16.92893218813456002 ) ) ;
#6876=ORIENTED_EDGE ( 'NONE', *, *, #8175, .T. ) ;
#6883=LINE ( 'NONE', #5284, #19807 ) ;
#6884=ADVANCED_FACE ( 'NONE', ( #2716 ), #1510, .T. ) ;
#6895=CARTESIAN_POINT ( 'NONE',  ( 203.3234976231972553, 23.93187681866832861, -14.00000000000004441 ) ) ;
#7002=VECTOR ( 'NONE', #6739, 1000.000000000000114 ) ;
#7003=EDGE_CURVE ( 'NONE', #10831, #13023, #8054, .T. ) ;
#7010=CARTESIAN_POINT ( 'NONE',  ( 184.9952905943350459, 3.535126980567737665, -6.000000000000071942 ) ) ;
#7036=( NAMED_UNIT ( * ) PLANE_ANGLE_UNIT ( ) SI_UNIT ( $, .RADIAN. ) );
#7123=DIRECTION ( 'NONE',  ( -0.8660254037844361541, -0.5000000000000042188, 0.000000000000000000 ) ) ;
#7129=DIRECTION ( 'NONE',  ( 0.5000000000000045519, -0.8660254037844360431, -4.006172263299080561E-16 ) ) ;
#7155=PLANE ( 'NONE',  #9639 ) ;
#7178=MECHANICAL_DESIGN_GEOMETRIC_PRESENTATION_REPRESENTATION('',(#19045),#7194);
#7194=( GEOMETRIC_REPRESENTATION_CONTEXT ( 3 ) GLOBAL_UNCERTAINTY_ASSIGNED_CONTEXT ( ( #12765 ) ) GLOBAL_UNIT_ASSIGNED_CONTEXT ( ( #19260, #1869, #5033 ) ) REPRESENTATION_CONTEXT ( 'NONE', 'WORKASPACE' ) );
#7255=CARTESIAN_POINT ( 'NONE',  ( 203.3234976231973405, 23.93187681866832861, -14.19648256269664621 ) ) ;
#7280=VERTEX_POINT ( 'NONE', #5708 ) ;
#7308=PLANE ( 'NONE',  #9931 ) ;
#7310=VECTOR ( 'NONE', #1341, 1000.000000000000114 ) ;
#7316=CARTESIAN_POINT ( 'NONE',  ( 216.3683575532814416, 33.19538101841234834, -14.00000000000004441 ) ) ;
#7338=CARTESIAN_POINT ( 'NONE',  ( 190.1694833127194499, 64.25747545832879837, -14.00000000000006395 ) ) ;
#7353=VERTEX_POINT ( 'NONE', #16121 ) ;
#7369=CARTESIAN_POINT ( 'NONE',  ( 193.9677224586705222, 21.99441912408888555, -14.00000000000005329 ) ) ;
#7384=CARTESIAN_POINT ( 'NONE',  ( 201.8742410413690322, 26.32933402587430294, -13.24682712576759158 ) ) ;
#7385=CARTESIAN_POINT ( 'NONE',  ( 182.3972143829817867, 2.035126980567750099, -6.000000000000071942 ) ) ;
#7425=FACE_OUTER_BOUND ( 'NONE', #4894, .T. ) ;
#7453=AXIS2_PLACEMENT_3D ( 'NONE', #16425, #1902, #11971 ) ;
#7464=LINE ( 'NONE', #12364, #17868 ) ;
#7481=LINE ( 'NONE', #9373, #15138 ) ;
#7500=PLANE ( 'NONE',  #7808 ) ;
#7502=ORIENTED_EDGE ( 'NONE', *, *, #10960, .F. ) ;
#7533=PRODUCT_CONTEXT ( 'NONE', #20702, 'mechanical' ) ;
#7551=CYLINDRICAL_SURFACE ( 'NONE', #17567, 4.999999999999975131 ) ;
#7570=ORIENTED_EDGE ( 'NONE', *, *, #12917, .F. ) ;
#7579=ADVANCED_FACE ( 'NONE', ( #8030 ), #18016, .T. ) ;
#7599=( BOUNDED_CURVE ( )  B_SPLINE_CURVE ( 3, ( #14663, #6875, #16433, #10045 ),
 .UNSPECIFIED., .F., .T. ) 
 B_SPLINE_CURVE_WITH_KNOTS ( ( 4, 4 ),
 ( 3.141592653589790451, 4.712388980384689674 ),
 .UNSPECIFIED. ) 
 CURVE ( )  GEOMETRIC_REPRESENTATION_ITEM ( )  RATIONAL_B_SPLINE_CURVE ( ( 1.000000000000000000, 0.8047378541243643824, 0.8047378541243643824, 1.000000000000000000 ) ) 
 REPRESENTATION_ITEM ( '' )  );
#7688=LINE ( 'NONE', #20417, #19174 ) ;
#7749=AXIS2_PLACEMENT_3D ( 'NONE', #13344, #9925, #16420 ) ;
#7759=CYLINDRICAL_SURFACE ( 'NONE', #3368, 15.00000000000001954 ) ;
#7781=CARTESIAN_POINT ( 'NONE',  ( 177.1791022559528983, 56.75747545832872731, -29.00000000000007105 ) ) ;
#7808=AXIS2_PLACEMENT_3D ( 'NONE', #11006, #17578, #17259 ) ;
#7845=EDGE_CURVE ( 'NONE', #15359, #3226, #15883, .T. ) ;
#7855=CARTESIAN_POINT ( 'NONE',  ( 211.0966947254765103, 27.85633560694163791, -15.52474636582213563 ) ) ;
#7904=CARTESIAN_POINT ( 'NONE',  ( 215.1183575532813848, 35.36044452787341186, -14.00000000000004441 ) ) ;
#7923=LINE ( 'NONE', #20546, #9711 ) ;
#7952=CARTESIAN_POINT ( 'NONE',  ( 209.1089911673190329, 31.29899458968461090, -15.52540737777744440 ) ) ;
#8030=FACE_OUTER_BOUND ( 'NONE', #9844, .T. ) ;
#8048=CARTESIAN_POINT ( 'NONE',  ( 208.9482664394169547, 31.70519001067595610, -14.65023073592818648 ) ) ;
#8054=LINE ( 'NONE', #14562, #363 ) ;
#8088=CARTESIAN_POINT ( 'NONE',  ( 208.9425382666943847, 31.71895361803450086, -13.34399656285678581 ) ) ;
#8098=ADVANCED_FACE ( 'NONE', ( #19875 ), #13642, .T. ) ;
#8101=CARTESIAN_POINT ( 'NONE',  ( 182.5734976231970563, 59.87193107572243633, -14.00000000000002842 ) ) ;
#8115=ADVANCED_FACE ( 'NONE', ( #11833 ), #18294, .F. ) ;
#8175=EDGE_CURVE ( 'NONE', #13077, #11736, #10542, .T. ) ;
#8188=CARTESIAN_POINT ( 'NONE',  ( 208.9194833127196489, 31.78152281641241572, -14.00000000000007816 ) ) ;
#8199=CARTESIAN_POINT ( 'NONE',  ( 211.4194833127196489, 27.45139579749023540, -14.00000000000004974 ) ) ;
#8222=EDGE_CURVE ( 'NONE', #7280, #14632, #20404, .T. ) ;
#8246=ORIENTED_EDGE ( 'NONE', *, *, #5886, .T. ) ;
#8260=DIRECTION ( 'NONE',  ( 0.5000000000000046629, -0.8660254037844360431, -4.006172263299081054E-16 ) ) ;
#8268=AXIS2_PLACEMENT_3D ( 'NONE', #6070, #8944, #9249 ) ;
#8326=ORIENTED_EDGE ( 'NONE', *, *, #10396, .F. ) ;
#8380=CARTESIAN_POINT ( 'NONE',  ( 202.5824069535873662, 24.78489278575215238, -12.54844597431177178 ) ) ;
#8393=LINE ( 'NONE', #14896, #3219 ) ;
#8400=CARTESIAN_POINT ( 'NONE',  ( 195.4677224586705222, 19.39634291273559086, -14.00000000000005329 ) ) ;
#8412=EDGE_CURVE ( 'NONE', #15359, #3430, #20842, .T. ) ;
#8446=CYLINDRICAL_SURFACE ( 'NONE', #20291, 2.499999999999994671 ) ;
#8447=CIRCLE ( 'NONE', #13541, 15.00000000000001954 ) ;
#8472=EDGE_CURVE ( 'NONE', #13077, #9607, #3392, .T. ) ;
#8486=CARTESIAN_POINT ( 'NONE',  ( 203.2866962553531778, 23.96679637293826204, -13.60843650710557462 ) ) ;
#8536=CARTESIAN_POINT ( 'NONE',  ( 202.5825078627354117, 24.78475806348888000, -15.45148755736461510 ) ) ;
#8560=ADVANCED_FACE ( 'NONE', ( #674 ), #6816, .T. ) ;
#8568=ORIENTED_EDGE ( 'NONE', *, *, #8994, .T. ) ;
#8575=CARTESIAN_POINT ( 'NONE',  ( 159.9952905943347901, 46.83639716978954226, -6.000000000000052403 ) ) ;
#8585=AXIS2_PLACEMENT_3D ( 'NONE', #18564, #4461, #17182 ) ;
#8615=DIRECTION ( 'NONE',  ( 0.5000000000000046629, -0.8660254037844360431, -4.006172263299081054E-16 ) ) ;
#8633=FACE_OUTER_BOUND ( 'NONE', #2272, .T. ) ;
#8637=CARTESIAN_POINT ( 'NONE',  ( 215.6183575532814416, 34.49441912408899924, -14.00000000000004441 ) ) ;
#8639=CARTESIAN_POINT ( 'NONE',  ( 201.9232846251233013, 26.15919357289564218, -14.99235525741147868 ) ) ;
#8652=LINE ( 'NONE', #2514, #10515 ) ;
#8676=VECTOR ( 'NONE', #12872, 1000.000000000000114 ) ;
#8682=DIRECTION ( 'NONE',  ( -0.8660254037844355990, -0.5000000000000051070, -2.294936594593527877E-16 ) ) ;
#8722=VECTOR ( 'NONE', #9201, 1000.000000000000000 ) ;
#8744=CARTESIAN_POINT ( 'NONE',  ( 203.2929909647774593, 23.96012768562937367, -14.39487826001324500 ) ) ;
#8745=CARTESIAN_POINT ( 'NONE',  ( 192.0123155716599683, 35.38128320186102371, -18.91295074164679235 ) ) ;
#8783=EDGE_LOOP ( 'NONE', ( #2433, #19629 ) ) ;
#8793=CIRCLE ( 'NONE', #11171, 2.499999999999994671 ) ;
#8806=CARTESIAN_POINT ( 'NONE',  ( 159.9952905943347901, 46.83639716978955647, -22.00000000000007816 ) ) ;
#8814=DIRECTION ( 'NONE',  ( -0.8660254037844360431, -0.5000000000000045519, -4.336808689942050277E-16 ) ) ;
#8821=EDGE_CURVE ( 'NONE', #7353, #10831, #12671, .T. ) ;
#8833=FACE_OUTER_BOUND ( 'NONE', #14181, .T. ) ;
#8879=EDGE_CURVE ( 'NONE', #9060, #3430, #4207, .T. ) ;
#8884=CARTESIAN_POINT ( 'NONE',  ( 203.2651618589191571, 23.98739702992933687, -13.51485263443600005 ) ) ;
#8904=DIRECTION ( 'NONE',  ( 0.5000000000000057732, -0.8660254037844353769, 0.000000000000000000 ) ) ;
#8905=AXIS2_PLACEMENT_3D ( 'NONE', #5920, #1071, #17178 ) ;
#8937=ORIENTED_EDGE ( 'NONE', *, *, #15027, .T. ) ;
#8944=DIRECTION ( 'NONE',  ( 0.5000000000000045519, -0.8660254037844360431, -4.006172263299080561E-16 ) ) ;
#8961=EDGE_LOOP ( 'NONE', ( #3778, #2335 ) ) ;
#8981=CARTESIAN_POINT ( 'NONE',  ( 202.4229321854107013, 25.03106559388957209, -12.49995495381715749 ) ) ;
#8994=EDGE_CURVE ( 'NONE', #15958, #10655, #2410, .T. ) ;
#9060=VERTEX_POINT ( 'NONE', #9705 ) ;
#9175=ORIENTED_EDGE ( 'NONE', *, *, #5295, .T. ) ;
#9179=LINE ( 'NONE', #20214, #4831 ) ;
#9201=DIRECTION ( 'NONE',  ( -7.930164461608272272E-15, -3.965082230804136136E-15, -1.000000000000000000 ) ) ;
#9218=ORIENTED_EDGE ( 'NONE', *, *, #20436, .T. ) ;
#9238=EDGE_CURVE ( 'NONE', #3756, #7280, #8652, .T. ) ;
#9249=DIRECTION ( 'NONE',  ( 0.8660254037844361541, 0.5000000000000043299, 0.000000000000000000 ) ) ;
#9253=AXIS2_PLACEMENT_3D ( 'NONE', #17512, #9322, #14244 ) ;
#9297=CARTESIAN_POINT ( 'NONE',  ( 184.9952905943350743, 3.535126980567765642, 0.9999999999999187317 ) ) ;
#9321=( BOUNDED_CURVE ( )  B_SPLINE_CURVE ( 3, ( #16364, #6375, #9567, #14376 ),
 .UNSPECIFIED., .F., .F. ) 
 B_SPLINE_CURVE_WITH_KNOTS ( ( 4, 4 ),
 ( 1.570796326794896558, 3.141592653589790451 ),
 .UNSPECIFIED. ) 
 CURVE ( )  GEOMETRIC_REPRESENTATION_ITEM ( )  RATIONAL_B_SPLINE_CURVE ( ( 1.000000000000000000, 0.8047378541243654926, 0.8047378541243654926, 1.000000000000000000 ) ) 
 REPRESENTATION_ITEM ( '' )  );
#9322=DIRECTION ( 'NONE',  ( 0.5000000000000046629, -0.8660254037844360431, -4.006172263299081054E-16 ) ) ;
#9323=EDGE_LOOP ( 'NONE', ( #9728, #16716 ) ) ;
#9332=VECTOR ( 'NONE', #14855, 1000.000000000000114 ) ;
#9365=DIRECTION ( 'NONE',  ( 0.5000000000000044409, -0.8660254037844360431, -4.006172263299080068E-16 ) ) ;
#9373=CARTESIAN_POINT ( 'NONE',  ( 184.9952905943350459, 3.535126980567737665, -6.000000000000071942 ) ) ;
#9461=CARTESIAN_POINT ( 'NONE',  ( 190.7433706042750146, 35.72129598111152404, -19.00000000000003908 ) ) ;
#9492=CARTESIAN_POINT ( 'NONE',  ( 173.9132435853527454, 54.87193107572242212, -14.00000000000002842 ) ) ;
#9511=EDGE_LOOP ( 'NONE', ( #12077, #12532, #1996, #19273 ) ) ;
#9512=ORIENTED_EDGE ( 'NONE', *, *, #4715, .F. ) ;
#9567=CARTESIAN_POINT ( 'NONE',  ( 183.9132435853528307, 37.55142300003366529, -11.07106781186552524 ) ) ;
#9568=ORIENTED_EDGE ( 'NONE', *, *, #16519, .F. ) ;
#9582=CARTESIAN_POINT ( 'NONE',  ( 211.2177619293863131, 27.70070338464699589, -12.73925315114813372 ) ) ;
#9601=EDGE_LOOP ( 'NONE', ( #20913, #18205 ) ) ;
#9607=VERTEX_POINT ( 'NONE', #14595 ) ;
#9614=ORIENTED_EDGE ( 'NONE', *, *, #6796, .T. ) ;
#9638=SHAPE_REPRESENTATION ( 'Drill Head Clamping Component', ( #18233 ), #2676 ) ;
#9639=AXIS2_PLACEMENT_3D ( 'NONE', #10644, #1019, #18825 ) ;
#9642=DIRECTION ( 'NONE',  ( 0.8660254037844360431, 0.5000000000000045519, 4.336808689942050277E-16 ) ) ;
#9646=CARTESIAN_POINT ( 'NONE',  ( 209.6747333788187291, 30.08054303420691866, -16.41975067815232947 ) ) ;
#9669=CARTESIAN_POINT ( 'NONE',  ( 194.0478494775925924, 31.85563505625661662, -14.00000000000006395 ) ) ;
#9687=CARTESIAN_POINT ( 'NONE',  ( 209.2403632168042975, 30.98959712955237578, -12.11805501175738620 ) ) ;
#9705=CARTESIAN_POINT ( 'NONE',  ( 191.0833833835253301, 36.99024094849632860, -9.087049258353282255 ) ) ;
#9711=VECTOR ( 'NONE', #4652, 1000.000000000000227 ) ;
#9728=ORIENTED_EDGE ( 'NONE', *, *, #4622, .F. ) ;
#9745=CARTESIAN_POINT ( 'NONE',  ( 208.9194833127196489, 31.78152281641241572, -14.00000000000007816 ) ) ;
#9754=EDGE_CURVE ( 'NONE', #15521, #18333, #2485, .T. ) ;
#9768=ORIENTED_EDGE ( 'NONE', *, *, #14613, .T. ) ;
#9777=DIRECTION ( 'NONE',  ( 0.5000000000000044409, -0.8660254037844360431, -4.006172263299080068E-16 ) ) ;
#9787=CARTESIAN_POINT ( 'NONE',  ( 210.6586702885180671, 28.45400361262161226, -11.82952947414952583 ) ) ;
#9844=EDGE_LOOP ( 'NONE', ( #10511, #13176, #14857, #12777 ) ) ;
#9867=FACE_OUTER_BOUND ( 'NONE', #2890, .T. ) ;
#9882=VERTEX_POINT ( 'NONE', #4383 ) ;
#9888=CARTESIAN_POINT ( 'NONE',  ( 210.3223930243060238, 28.95850756564502859, -11.57946969169901763 ) ) ;
#9921=CARTESIAN_POINT ( 'NONE',  ( 157.3972143829815309, 45.33639716978955647, -6.000000000000052403 ) ) ;
#9925=DIRECTION ( 'NONE',  ( -0.8660254037844360431, -0.5000000000000045519, -4.336808689942050277E-16 ) ) ;
#9931=AXIS2_PLACEMENT_3D ( 'NONE', #12204, #5924, #18776 ) ;
#9934=LINE ( 'NONE', #11543, #9332 ) ;
#9954=CARTESIAN_POINT ( 'NONE',  ( 203.0967589511048743, 24.15675494531242506, -13.08406428195295668 ) ) ;
#9962=DIRECTION ( 'NONE',  ( 0.5000000000000044409, -0.8660254037844360431, -4.006172263299080068E-16 ) ) ;
#10045=CARTESIAN_POINT ( 'NONE',  ( 190.7433706042750146, 35.72129598111152404, -19.00000000000003908 ) ) ;
#10108=FACE_OUTER_BOUND ( 'NONE', #12349, .T. ) ;
#10184=CARTESIAN_POINT ( 'NONE',  ( 202.1791022559531541, 13.45620526910692227, -29.00000000000009237 ) ) ;
#10192=LINE ( 'NONE', #8400, #17882 ) ;
#10196=DIRECTION ( 'NONE',  ( 0.5000000000000044409, -0.8660254037844360431, -4.006172263299080068E-16 ) ) ;
#10320=CARTESIAN_POINT ( 'NONE',  ( 202.1920911364529445, 25.46077609459828750, -15.45182294182971283 ) ) ;
#10345=CARTESIAN_POINT ( 'NONE',  ( 157.3972143829815309, 45.33639716978955647, -6.000000000000052403 ) ) ;
#10393=EDGE_LOOP ( 'NONE', ( #3773, #5426, #11201, #6592 ) ) ;
#10396=EDGE_CURVE ( 'NONE', #10601, #14228, #4002, .T. ) ;
#10405=VECTOR ( 'NONE', #18445, 1000.000000000000000 ) ;
#10458=CARTESIAN_POINT ( 'NONE',  ( 203.3234976231973405, 23.93187681866833216, -13.90173226369915405 ) ) ;
#10465=LINE ( 'NONE', #8575, #12889 ) ;
#10495=VECTOR ( 'NONE', #9365, 1000.000000000000114 ) ;
#10511=ORIENTED_EDGE ( 'NONE', *, *, #11959, .F. ) ;
#10515=VECTOR ( 'NONE', #18517, 1000.000000000000114 ) ;
#10542=LINE ( 'NONE', #17028, #18966 ) ;
#10550=CARTESIAN_POINT ( 'NONE',  ( 177.1791022559528983, 56.75747545832872731, -14.00000000000006395 ) ) ;
#10575=CARTESIAN_POINT ( 'NONE',  ( 202.6368254117890046, 24.70800346662761626, -12.57697892669095019 ) ) ;
#10601=VERTEX_POINT ( 'NONE', #14401 ) ;
#10608=AXIS2_PLACEMENT_3D ( 'NONE', #16985, #8814, #10610 ) ;
#10610=DIRECTION ( 'NONE',  ( 0.5000000000000057732, -0.8660254037844353769, 0.000000000000000000 ) ) ;
#10628=CARTESIAN_POINT ( 'NONE',  ( 159.9952905943348469, 46.83639716978957068, 0.9999999999999386047 ) ) ;
#10635=MANIFOLD_SOLID_BREP ( 'Cut-Extrude8', #5927 ) ;
#10640=CARTESIAN_POINT ( 'NONE',  ( 159.9952905943347901, 46.83639716978955647, -22.00000000000007816 ) ) ;
#10644=CARTESIAN_POINT ( 'NONE',  ( 177.1791022559528983, 56.75747545832873442, -29.00000000000007105 ) ) ;
#10655=VERTEX_POINT ( 'NONE', #8101 ) ;
#10660=DIRECTION ( 'NONE',  ( -0.8660254037844360431, -0.5000000000000045519, -4.336808689942049784E-16 ) ) ;
#10698=ORIENTED_EDGE ( 'NONE', *, *, #861, .T. ) ;
#10725=CARTESIAN_POINT ( 'NONE',  ( 159.9952905943348469, 46.83639716978957068, 0.9999999999999386047 ) ) ;
#10740=ORIENTED_EDGE ( 'NONE', *, *, #11597, .F. ) ;
#10754=ORIENTED_EDGE ( 'NONE', *, *, #12917, .T. ) ;
#10831=VERTEX_POINT ( 'NONE', #1339 ) ;
#10871=CARTESIAN_POINT ( 'NONE',  ( 184.9952905943350459, 3.535126980567751431, -22.00000000000009948 ) ) ;
#10904=ORIENTED_EDGE ( 'NONE', *, *, #20392, .F. ) ;
#10946=FACE_OUTER_BOUND ( 'NONE', #9323, .T. ) ;
#10954=CARTESIAN_POINT ( 'NONE',  ( 202.1791022559531541, 13.45620526910691694, -14.00000000000008527 ) ) ;
#10960=EDGE_CURVE ( 'NONE', #11736, #15521, #12145, .T. ) ;
#10994=B_SPLINE_CURVE_WITH_KNOTS ( 'NONE', 3,
 ( #6455, #13058, #17826, #15827, #12959, #11144, #17409, #7855, #19407, #17729, #1300, #3193, #20682, #4886, #1504, #16140, #3295, #9646, #6356, #2888, #14249, #6155, #16043, #1607, #7952, #11353, #12851, #14354, #8048, #19305, #3097, #9745 ),
 .UNSPECIFIED., .F., .F.,
 ( 4, 2, 2, 2, 2, 2, 2, 2, 2, 2, 2, 2, 2, 2, 2, 4 ),
 ( 5.204170427930421283E-18, 0.0004893630623245339177, 0.0009787261246490626312, 0.001468089186973591236, 0.001957452249298120058, 0.002936178373947171197, 0.003425541436271701320, 0.003914904498596230575, 0.004404267560920760265, 0.004893630623245289954, 0.005382993685569818776, 0.005872356747894348465, 0.006361719810218879022, 0.006851082872543407844, 0.007340445934867937533, 0.007829808997192468090 ),
 .UNSPECIFIED. ) ;
#11006=CARTESIAN_POINT ( 'NONE',  ( 157.3972143829815309, 45.33639716978955647, -6.000000000000052403 ) ) ;
#11014=EDGE_LOOP ( 'NONE', ( #6837, #5798, #946, #9768 ) ) ;
#11050=LINE ( 'NONE', #4584, #2811 ) ;
#11058=FACE_OUTER_BOUND ( 'NONE', #17587, .T. ) ;
#11131=ORIENTED_EDGE ( 'NONE', *, *, #263, .F. ) ;
#11144=CARTESIAN_POINT ( 'NONE',  ( 211.2576524688788311, 27.65102446918777090, -15.10969539796795580 ) ) ;
#11171=AXIS2_PLACEMENT_3D ( 'NONE', #12055, #18519, #20101 ) ;
#11182=CARTESIAN_POINT ( 'NONE',  ( 216.3683575532813848, 33.19538101841231992, -14.00000000000004441 ) ) ;
#11187=ORIENTED_EDGE ( 'NONE', *, *, #20050, .F. ) ;
#11188=CARTESIAN_POINT ( 'NONE',  ( 210.1532566776551789, 29.23042781764359432, -11.51600929819806396 ) ) ;
#11201=ORIENTED_EDGE ( 'NONE', *, *, #9238, .T. ) ;
#11221=ADVANCED_FACE ( 'NONE', ( #4180 ), #12456, .T. ) ;
#11227=ORIENTED_EDGE ( 'NONE', *, *, #16519, .T. ) ;
#11231=VECTOR ( 'NONE', #3710, 1000.000000000000114 ) ;
#11265=CARTESIAN_POINT ( 'NONE',  ( 191.5478494775925640, 36.18576207517880050, -14.00000000000006395 ) ) ;
#11353=CARTESIAN_POINT ( 'NONE',  ( 209.0403034353200269, 31.46832416448081560, -15.25488430973097209 ) ) ;
#11398=DIRECTION ( 'NONE',  ( 0.5000000000000044409, -0.8660254037844360431, 0.000000000000000000 ) ) ;
#11455=ORIENTED_EDGE ( 'NONE', *, *, #8222, .F. ) ;
#11495=CARTESIAN_POINT ( 'NONE',  ( 209.6021936215576034, 30.22200596923644511, -11.62851498981274290 ) ) ;
#11543=CARTESIAN_POINT ( 'NONE',  ( 189.0478494775925355, 40.51588909410097727, -14.00000000000006395 ) ) ;
#11561=ORIENTED_EDGE ( 'NONE', *, *, #8412, .F. ) ;
#11567=DIRECTION ( 'NONE',  ( -0.8660254037844360431, -0.5000000000000045519, -4.336808689942049784E-16 ) ) ;
#11575=CARTESIAN_POINT ( 'NONE',  ( 190.9712048706970791, 36.57158503910370939, -9.029101044830413869 ) ) ;
#11597=EDGE_CURVE ( 'NONE', #4012, #14531, #2817, .T. ) ;
#11602=CARTESIAN_POINT ( 'NONE',  ( 190.7433706042750146, 35.72129598111152404, -9.000000000000062172 ) ) ;
#11626=DIRECTION ( 'NONE',  ( 2.003086131649568876E-16, -3.469446951953589044E-16, 1.000000000000000000 ) ) ;
#11644=ORIENTED_EDGE ( 'NONE', *, *, #20787, .F. ) ;
#11680=CARTESIAN_POINT ( 'NONE',  ( 202.8019581880755595, 24.48753073112860079, -12.69065112601704293 ) ) ;
#11687=ORIENTED_EDGE ( 'NONE', *, *, #16037, .T. ) ;
#11689=LINE ( 'NONE', #11794, #14123 ) ;
#11709=VERTEX_POINT ( 'NONE', #19530 ) ;
#11736=VERTEX_POINT ( 'NONE', #8188 ) ;
#11750=EDGE_CURVE ( 'NONE', #12839, #15359, #15617, .T. ) ;
#11762=ORIENTED_EDGE ( 'NONE', *, *, #962, .F. ) ;
#11794=CARTESIAN_POINT ( 'NONE',  ( 157.3972143829815309, 45.33639716978957068, -22.00000000000007816 ) ) ;
#11800=ORIENTED_EDGE ( 'NONE', *, *, #16516, .F. ) ;
#11829=CARTESIAN_POINT ( 'NONE',  ( 202.0445642045415582, 25.79900422344375599, -15.30999104003096889 ) ) ;
#11833=FACE_OUTER_BOUND ( 'NONE', #18232, .T. ) ;
#11848=ORIENTED_EDGE ( 'NONE', *, *, #1129, .T. ) ;
#11873=AXIS2_PLACEMENT_3D ( 'NONE', #7316, #3828, #5715 ) ;
#11938=CYLINDRICAL_SURFACE ( 'NONE', #2571, 1.499999999999990896 ) ;
#11940=CARTESIAN_POINT ( 'NONE',  ( 201.8620183822125398, 26.37541784318060678, -14.66741346640867150 ) ) ;
#11957=CARTESIAN_POINT ( 'NONE',  ( 177.1791022559528983, 56.75747545832872731, -14.00000000000006395 ) ) ;
#11959=EDGE_CURVE ( 'NONE', #19623, #2860, #2053, .T. ) ;
#11971=DIRECTION ( 'NONE',  ( 0.000000000000000000, 1.000000000000000000, 3.469446951953589044E-16 ) ) ;
#11983=ORIENTED_EDGE ( 'NONE', *, *, #16091, .F. ) ;
#12042=CARTESIAN_POINT ( 'NONE',  ( 202.4761207370255818, 24.94531058701918980, -15.49001580682321233 ) ) ;
#12046=CARTESIAN_POINT ( 'NONE',  ( 202.1791022559531541, 13.45620526910691694, 0.9999999999999232836 ) ) ;
#12055=CARTESIAN_POINT ( 'NONE',  ( 216.3683575532813848, 33.19538101841231992, -14.00000000000004441 ) ) ;
#12077=ORIENTED_EDGE ( 'NONE', *, *, #8175, .F. ) ;
#12145=B_SPLINE_CURVE_WITH_KNOTS ( 'NONE', 3,
 ( #20822, #12892, #8088, #6297, #18073, #17873, #4717, #9687, #12789, #16181, #3137, #11495, #3338, #14495, #15978, #20921, #11188, #9888, #14394, #14599, #9787, #1649, #16272, #6601, #9582, #1752, #16081, #19249, #6705, #8199 ),
 .UNSPECIFIED., .F., .F.,
 ( 4, 2, 2, 2, 2, 2, 2, 2, 2, 2, 2, 2, 2, 2, 4 ),
 ( 0.007829808997192468090, 0.008808290957735770768, 0.009297531938007422975, 0.009786772918279073447, 0.01027601389855072565, 0.01076525487882237613, 0.01125449585909402833, 0.01174373683936567880, 0.01223297781963733101, 0.01272221879990898322, 0.01321145978018063369, 0.01370070076045228416, 0.01467918272099555388, 0.01516842370126719915, 0.01565766468153884441 ),
 .UNSPECIFIED. ) ;
#12153=FACE_OUTER_BOUND ( 'NONE', #10393, .T. ) ;
#12204=CARTESIAN_POINT ( 'NONE',  ( 202.1791022559531541, 13.45620526910691694, -14.00000000000008527 ) ) ;
#12220=EDGE_CURVE ( 'NONE', #9607, #15521, #11050, .T. ) ;
#12224=CIRCLE ( 'NONE', #11873, 1.499999999999993783 ) ;
#12295=FACE_OUTER_BOUND ( 'NONE', #15305, .T. ) ;
#12339=CARTESIAN_POINT ( 'NONE',  ( 184.9952905943350743, 3.535126980567765642, 0.9999999999999187317 ) ) ;
#12349=EDGE_LOOP ( 'NONE', ( #6541, #16720, #15098, #465 ) ) ;
#12364=CARTESIAN_POINT ( 'NONE',  ( 179.0478494775924503, 57.83639716978969147, -9.087049258353273373 ) ) ;
#12378=LINE ( 'NONE', #7369, #7310 ) ;
#12424=FACE_BOUND ( 'NONE', #15647, .T. ) ;
#12444=CARTESIAN_POINT ( 'NONE',  ( 216.3683575532813848, 33.19538101841231992, -14.00000000000004441 ) ) ;
#12452=CARTESIAN_POINT ( 'NONE',  ( 182.3972143829817867, 2.035126980567750099, -6.000000000000071942 ) ) ;
#12456=PLANE ( 'NONE',  #6129 ) ;
#12509=ADVANCED_FACE ( 'NONE', ( #6666 ), #19605, .F. ) ;
#12532=ORIENTED_EDGE ( 'NONE', *, *, #8472, .T. ) ;
#12566=ADVANCED_FACE ( 'NONE', ( #13896 ), #17390, .T. ) ;
#12606=ORIENTED_EDGE ( 'NONE', *, *, #15085, .F. ) ;
#12638=CARTESIAN_POINT ( 'NONE',  ( 188.9132435853528591, 28.89116896218935082, -14.00000000000004086 ) ) ;
#12671=B_SPLINE_CURVE_WITH_KNOTS ( 'NONE', 3,
 ( #450, #939, #2536, #1934, #13376, #19722, #7384, #837, #20328, #5294, #19827, #4009, #5193, #8981, #15384, #8380, #10575, #11680, #18143, #5799, #9954, #15583, #339, #8884, #8486, #16945, #10458, #6895 ),
 .UNSPECIFIED., .F., .F.,
 ( 4, 2, 2, 2, 2, 2, 2, 2, 2, 2, 2, 2, 2, 4 ),
 ( 3.469446951953614189E-18, 0.0002948126770087786098, 0.0005896253540175537501, 0.0008844380310263289446, 0.001179250708035104031, 0.001768876062052661575, 0.002358501416070219337, 0.002653314093078998435, 0.002948126770087776665, 0.003537752124105387769, 0.003832564801114191587, 0.004127377478122994971, 0.004422190155131798354, 0.004717002832140601738 ),
 .UNSPECIFIED. ) ;
#12765=UNCERTAINTY_MEASURE_WITH_UNIT (LENGTH_MEASURE( 1.000000000000000082E-05 ), #19260, 'distance_accuracy_value', 'NONE');
#12777=ORIENTED_EDGE ( 'NONE', *, *, #6374, .T. ) ;
#12789=CARTESIAN_POINT ( 'NONE',  ( 209.2925290576059467, 30.87145858698718826, -12.01256274262992463 ) ) ;
#12810=ORIENTED_EDGE ( 'NONE', *, *, #5014, .F. ) ;
#12839=VERTEX_POINT ( 'NONE', #521 ) ;
#12851=CARTESIAN_POINT ( 'NONE',  ( 209.0112450435238145, 31.54208512462550118, -15.10854341765127806 ) ) ;
#12856=LINE ( 'NONE', #10640, #709 ) ;
#12860=ORIENTED_EDGE ( 'NONE', *, *, #1129, .F. ) ;
#12872=DIRECTION ( 'NONE',  ( -0.8660254037844360431, -0.5000000000000044409, -4.336808689942049290E-16 ) ) ;
#12889=VECTOR ( 'NONE', #15179, 1000.000000000000114 ) ;
#12892=CARTESIAN_POINT ( 'NONE',  ( 208.9194833127196489, 31.78152281641241572, -13.67345714572792659 ) ) ;
#12917=EDGE_CURVE ( 'NONE', #10655, #7353, #9179, .T. ) ;
#12959=CARTESIAN_POINT ( 'NONE',  ( 211.3372400686716617, 27.55192669161114694, -14.80705122880212166 ) ) ;
#13001=CARTESIAN_POINT ( 'NONE',  ( 159.9952905943347901, 46.83639716978954226, -6.000000000000052403 ) ) ;
#13023=VERTEX_POINT ( 'NONE', #2635 ) ;
#13040=ORIENTED_EDGE ( 'NONE', *, *, #8412, .T. ) ;
#13058=CARTESIAN_POINT ( 'NONE',  ( 211.4194833127197342, 27.45139579749024605, -14.16549164512199965 ) ) ;
#13077=VERTEX_POINT ( 'NONE', #7904 ) ;
#13142=PRODUCT_DEFINITION ( 'UNKNOWN', '', #19263, #15547 ) ;
#13176=ORIENTED_EDGE ( 'NONE', *, *, #861, .F. ) ;
#13178=ADVANCED_FACE ( 'NONE', ( #10108 ), #13215, .T. ) ;
#13215=PLANE ( 'NONE',  #20089 ) ;
#13226=AXIS2_PLACEMENT_3D ( 'NONE', #11265, #13846, #17735 ) ;
#13259=ADVANCED_FACE ( 'NONE', ( #5443, #10946 ), #20580, .F. ) ;
#13331=ORIENTED_EDGE ( 'NONE', *, *, #20883, .F. ) ;
#13344=CARTESIAN_POINT ( 'NONE',  ( 191.5478494775925640, 36.18576207517880050, -14.00000000000006395 ) ) ;
#13350=EDGE_CURVE ( 'NONE', #14531, #16924, #4485, .T. ) ;
#13361=LINE ( 'NONE', #6553, #14817 ) ;
#13369=CARTESIAN_POINT ( 'NONE',  ( 157.3972143829815309, 45.33639716978957068, -22.00000000000007816 ) ) ;
#13376=CARTESIAN_POINT ( 'NONE',  ( 201.8424605768971389, 26.45147170171050277, -13.51420023870525711 ) ) ;
#13415=( LENGTH_UNIT ( ) NAMED_UNIT ( * ) SI_UNIT ( .MILLI., .METRE. ) );
#13424=AXIS2_PLACEMENT_3D ( 'NONE', #11957, #716, #5781 ) ;
#13425=CARTESIAN_POINT ( 'NONE',  ( 201.8234976231972553, 26.52995303002161265, -14.09970077338581973 ) ) ;
#13445=VECTOR ( 'NONE', #17818, 1000.000000000000000 ) ;
#13524=FACE_OUTER_BOUND ( 'NONE', #14988, .T. ) ;
#13541=AXIS2_PLACEMENT_3D ( 'NONE', #10954, #1311, #19318 ) ;
#13587=DIRECTION ( 'NONE',  ( 0.8660254037844344888, 0.5000000000000069944, 0.000000000000000000 ) ) ;
#13601=ORIENTED_EDGE ( 'NONE', *, *, #13350, .F. ) ;
#13608=DIRECTION ( 'NONE',  ( 0.8660254037844355990, 0.5000000000000051070, -1.748523119690306661E-16 ) ) ;
#13621=CARTESIAN_POINT ( 'NONE',  ( 178.2433706042749009, 57.37193107572242923, -14.00000000000002842 ) ) ;
#13638=CARTESIAN_POINT ( 'NONE',  ( 203.0529676813258106, 24.20295447737667516, -14.99132954693030229 ) ) ;
#13642=CYLINDRICAL_SURFACE ( 'NONE', #6742, 2.499999999999994671 ) ;
#13696=ADVANCED_FACE ( 'NONE', ( #15605, #20457 ), #7308, .F. ) ;
#13707=ADVANCED_FACE ( 'NONE', ( #12424, #17082 ), #1074, .T. ) ;
#13738=CARTESIAN_POINT ( 'NONE',  ( 202.2784612918522100, 25.28746711354437693, -15.49033546657680915 ) ) ;
#13771=AXIS2_PLACEMENT_3D ( 'NONE', #4598, #19327, #17536 ) ;
#13782=CARTESIAN_POINT ( 'NONE',  ( 211.4194833127196489, 27.45139579749023540, -14.00000000000004974 ) ) ;
#13843=CARTESIAN_POINT ( 'NONE',  ( 194.7177224586705222, 20.69538101841223821, -14.00000000000005329 ) ) ;
#13846=DIRECTION ( 'NONE',  ( -0.8660254037844361541, -0.5000000000000045519, -4.336808689942050770E-16 ) ) ;
#13847=DIRECTION ( 'NONE',  ( 0.5000000000000044409, -0.8660254037844360431, -4.006172263299080068E-16 ) ) ;
#13884=CARTESIAN_POINT ( 'NONE',  ( 190.1694833127194499, 64.25747545832879837, -14.00000000000006395 ) ) ;
#13896=FACE_OUTER_BOUND ( 'NONE', #8783, .T. ) ;
#13898=AXIS2_PLACEMENT_3D ( 'NONE', #11182, #17662, #6389 ) ;
#13916=DIRECTION ( 'NONE',  ( 0.5000000000000046629, -0.8660254037844360431, -4.006172263299081054E-16 ) ) ;
#13938=VERTEX_POINT ( 'NONE', #1691 ) ;
#14023=EDGE_CURVE ( 'NONE', #270, #11709, #9934, .T. ) ;
#14025=AXIS2_PLACEMENT_3D ( 'NONE', #219, #5076, #14974 ) ;
#14029=DIRECTION ( 'NONE',  ( 0.8660254037844358210, 0.5000000000000047740, 0.000000000000000000 ) ) ;
#14030=ORIENTED_EDGE ( 'NONE', *, *, #4622, .T. ) ;
#14036=DIRECTION ( 'NONE',  ( -0.8660254037844361541, -0.5000000000000045519, -4.336808689942050770E-16 ) ) ;
#14044=DIRECTION ( 'NONE',  ( 0.8660254037844361541, 0.5000000000000043299, 0.000000000000000000 ) ) ;
#14123=VECTOR ( 'NONE', #9962, 1000.000000000000114 ) ;
#14181=EDGE_LOOP ( 'NONE', ( #3762, #2462, #10754, #19168, #14341, #6195, #5170, #13040, #4884, #11187, #18850, #15344 ) ) ;
#14228=VERTEX_POINT ( 'NONE', #4323 ) ;
#14233=ORIENTED_EDGE ( 'NONE', *, *, #19751, .F. ) ;
#14244=DIRECTION ( 'NONE',  ( 0.8660254037844354880, 0.5000000000000053291, 0.000000000000000000 ) ) ;
#14249=CARTESIAN_POINT ( 'NONE',  ( 209.4061049964370227, 30.62402206602542165, -16.16870873105882112 ) ) ;
#14251=VECTOR ( 'NONE', #1459, 1000.000000000000114 ) ;
#14253=DIRECTION ( 'NONE',  ( -0.5000000000000034417, 0.8660254037844364872, 0.000000000000000000 ) ) ;
#14256=DIRECTION ( 'NONE',  ( -0.8660254037844355990, -0.5000000000000051070, -2.294936594593527877E-16 ) ) ;
#14273=LINE ( 'NONE', #9669, #8676 ) ;
#14322=EDGE_LOOP ( 'NONE', ( #14030, #6876, #601, #1702 ) ) ;
#14326=VECTOR ( 'NONE', #16623, 1000.000000000000114 ) ;
#14341=ORIENTED_EDGE ( 'NONE', *, *, #7003, .T. ) ;
#14354=CARTESIAN_POINT ( 'NONE',  ( 208.9653092665176644, 31.66033285536642339, -14.80609056993748140 ) ) ;
#14362=CARTESIAN_POINT ( 'NONE',  ( 192.0123155716598262, 35.38128320186126530, -9.087049258353282255 ) ) ;
#14376=CARTESIAN_POINT ( 'NONE',  ( 183.9132435853528307, 37.55142300003367950, -14.00000000000003730 ) ) ;
#14392=ORIENTED_EDGE ( 'NONE', *, *, #5014, .T. ) ;
#14394=CARTESIAN_POINT ( 'NONE',  ( 210.4088278365934457, 28.82459569483809503, -11.62765399154570289 ) ) ;
#14401=CARTESIAN_POINT ( 'NONE',  ( 192.0123155716599683, 35.38128320186102371, -18.91295074164679235 ) ) ;
#14458=ORIENTED_EDGE ( 'NONE', *, *, #8994, .F. ) ;
#14495=CARTESIAN_POINT ( 'NONE',  ( 209.8252572024504445, 29.79871034852264344, -11.51651525544093602 ) ) ;
#14497=FACE_OUTER_BOUND ( 'NONE', #11014, .T. ) ;
#14501=APPLICATION_CONTEXT ( 'automotive_design' ) ;
#14519=CARTESIAN_POINT ( 'NONE',  ( 178.2433706042749009, 57.37193107572242923, -14.00000000000002842 ) ) ;
#14531=VERTEX_POINT ( 'NONE', #12046 ) ;
#14532=LINE ( 'NONE', #9921, #7002 ) ;
#14546=CIRCLE ( 'NONE', #7749, 5.000000000000002665 ) ;
#14562=CARTESIAN_POINT ( 'NONE',  ( 182.5734976231970563, 59.87193107572243633, -14.00000000000002842 ) ) ;
#14582=ADVANCED_FACE ( 'NONE', ( #12153 ), #7155, .T. ) ;
#14595=CARTESIAN_POINT ( 'NONE',  ( 217.6183575532813848, 31.03031750895123864, -14.00000000000004441 ) ) ;
#14599=CARTESIAN_POINT ( 'NONE',  ( 210.5768882188229725, 28.57253264919412672, -11.75286491306098924 ) ) ;
#14613=EDGE_CURVE ( 'NONE', #3756, #13938, #462, .T. ) ;
#14632=VERTEX_POINT ( 'NONE', #10184 ) ;
#14649=CIRCLE ( 'NONE', #5462, 15.00000000000001954 ) ;
#14663=CARTESIAN_POINT ( 'NONE',  ( 183.9132435853528307, 37.55142300003367950, -14.00000000000003730 ) ) ;
#14700=EDGE_CURVE ( 'NONE', #13938, #14632, #8393, .T. ) ;
#14726=ORIENTED_EDGE ( 'NONE', *, *, #15085, .T. ) ;
#14741=ORIENTED_EDGE ( 'NONE', *, *, #16037, .F. ) ;
#14808=ORIENTED_EDGE ( 'NONE', *, *, #11959, .T. ) ;
#14817=VECTOR ( 'NONE', #16225, 1000.000000000000114 ) ;
#14855=DIRECTION ( 'NONE',  ( -0.8660254037844360431, -0.5000000000000044409, -4.336808689942049290E-16 ) ) ;
#14857=ORIENTED_EDGE ( 'NONE', *, *, #19751, .T. ) ;
#14886=EDGE_CURVE ( 'NONE', #15521, #11736, #10994, .T. ) ;
#14896=CARTESIAN_POINT ( 'NONE',  ( 202.1791022559531541, 13.45620526910692938, -29.00000000000009237 ) ) ;
#14904=DIRECTION ( 'NONE',  ( 0.8660254037844361541, 0.5000000000000044409, 0.000000000000000000 ) ) ;
#14921=CARTESIAN_POINT ( 'NONE',  ( 203.3234976231972553, 23.93187681866832861, -14.00000000000004441 ) ) ;
#14943=AXIS2_PLACEMENT_3D ( 'NONE', #14519, #3047, #17577 ) ;
#14974=DIRECTION ( 'NONE',  ( 0.8660254037844358210, 0.5000000000000047740, 0.000000000000000000 ) ) ;
#14976=VERTEX_POINT ( 'NONE', #19921 ) ;
#14980=LINE ( 'NONE', #13369, #16115 ) ;
#14988=EDGE_LOOP ( 'NONE', ( #1988, #16562, #16694, #11848 ) ) ;
#14992=CARTESIAN_POINT ( 'NONE',  ( 190.8575367324608010, 36.14736977200433898, -9.000000000000063949 ) ) ;
#15027=EDGE_CURVE ( 'NONE', #2860, #13938, #6883, .T. ) ;
#15030=CYLINDRICAL_SURFACE ( 'NONE', #18097, 5.000000000000002665 ) ;
#15037=CARTESIAN_POINT ( 'NONE',  ( 202.6369081707363193, 24.70788110947296445, -15.42298940083595227 ) ) ;
#15043=EDGE_LOOP ( 'NONE', ( #14726, #2937, #15977, #6142, #17785, #11455 ) ) ;
#15085=EDGE_CURVE ( 'NONE', #7280, #15664, #2568, .T. ) ;
#15098=ORIENTED_EDGE ( 'NONE', *, *, #16894, .T. ) ;
#15138=VECTOR ( 'NONE', #17355, 1000.000000000000227 ) ;
#15139=CARTESIAN_POINT ( 'NONE',  ( 202.1519482485907986, 25.54804868556654185, -15.42265203330069490 ) ) ;
#15179=DIRECTION ( 'NONE',  ( 0.5000000000000044409, -0.8660254037844360431, -4.006172263299080068E-16 ) ) ;
#15220=CARTESIAN_POINT ( 'NONE',  ( 159.9952905943348469, 46.83639716978958489, -29.00000000000006750 ) ) ;
#15242=CARTESIAN_POINT ( 'NONE',  ( 203.1748089687253582, 24.07645447784576831, -14.75390691332407300 ) ) ;
#15305=EDGE_LOOP ( 'NONE', ( #2611, #19095, #2482, #10698 ) ) ;
#15332=DIRECTION ( 'NONE',  ( 0.5000000000000045519, -0.8660254037844360431, -4.006172263299080561E-16 ) ) ;
#15344=ORIENTED_EDGE ( 'NONE', *, *, #723, .T. ) ;
#15350=CARTESIAN_POINT ( 'NONE',  ( 201.8234976231972553, 26.52995303002162331, -14.00000000000004619 ) ) ;
#15359=VERTEX_POINT ( 'NONE', #12638 ) ;
#15384=CARTESIAN_POINT ( 'NONE',  ( 202.4756851904152484, 24.94598553735895763, -12.50985653407239795 ) ) ;
#15513=ORIENTED_EDGE ( 'NONE', *, *, #15580, .T. ) ;
#15521=VERTEX_POINT ( 'NONE', #13782 ) ;
#15531=CIRCLE ( 'NONE', #16535, 4.999999999999976907 ) ;
#15539=LINE ( 'NONE', #12452, #18229 ) ;
#15547=PRODUCT_DEFINITION_CONTEXT ( 'detailed design', #14501, 'design' ) ;
#15580=EDGE_CURVE ( 'NONE', #4012, #14976, #20228, .T. ) ;
#15583=CARTESIAN_POINT ( 'NONE',  ( 203.1748324726931401, 24.07643182039328877, -13.24616221489253576 ) ) ;
#15594=ORIENTED_EDGE ( 'NONE', *, *, #4367, .T. ) ;
#15604=AXIS2_PLACEMENT_3D ( 'NONE', #20171, #7129, #14904 ) ;
#15605=FACE_BOUND ( 'NONE', #9601, .T. ) ;
#15617=( BOUNDED_CURVE ( )  B_SPLINE_CURVE ( 3, ( #9461, #20909, #1434, #17957 ),
 .UNSPECIFIED., .F., .T. ) 
 B_SPLINE_CURVE_WITH_KNOTS ( ( 4, 4 ),
 ( 4.712388980384689674, 6.283185307179586232 ),
 .UNSPECIFIED. ) 
 CURVE ( )  GEOMETRIC_REPRESENTATION_ITEM ( )  RATIONAL_B_SPLINE_CURVE ( ( 1.000000000000000000, 0.8047378541243649375, 0.8047378541243649375, 1.000000000000000000 ) ) 
 REPRESENTATION_ITEM ( '' )  );
#15625=CARTESIAN_POINT ( 'NONE',  ( 191.5478494775925640, 36.18576207517880050, -14.00000000000006395 ) ) ;
#15647=EDGE_LOOP ( 'NONE', ( #778, #8568 ) ) ;
#15659=CARTESIAN_POINT ( 'NONE',  ( 191.1694443951678863, 35.60712985292571631, -19.00000000000003908 ) ) ;
#15661=CARTESIAN_POINT ( 'NONE',  ( 190.7433706042750146, 35.72129598111152404, -9.000000000000062172 ) ) ;
#15664=VERTEX_POINT ( 'NONE', #13884 ) ;
#15686=DIRECTION ( 'NONE',  ( 0.5000000000000044409, -0.8660254037844360431, -4.006172263299080068E-16 ) ) ;
#15745=ORIENTED_EDGE ( 'NONE', *, *, #16516, .T. ) ;
#15827=CARTESIAN_POINT ( 'NONE',  ( 211.3681101147246011, 27.51407081612045857, -14.64810036304597496 ) ) ;
#15852=DIRECTION ( 'NONE',  ( 0.5000000000000044409, -0.8660254037844360431, -4.006172263299080068E-16 ) ) ;
#15854=( BOUNDED_CURVE ( )  B_SPLINE_CURVE ( 3, ( #3104, #20581, #6054, #14362 ),
 .UNSPECIFIED., .F., .F. ) 
 B_SPLINE_CURVE_WITH_KNOTS ( ( 4, 4 ),
 ( 4.712388980384689674, 4.899261154233307991 ),
 .UNSPECIFIED. ) 
 CURVE ( )  GEOMETRIC_REPRESENTATION_ITEM ( )  RATIONAL_B_SPLINE_CURVE ( ( 1.000000000000000000, 0.9970920157757060531, 0.9970920157757060531, 1.000000000000000000 ) ) 
 REPRESENTATION_ITEM ( '' )  );
#15883=LINE ( 'NONE', #9492, #14251 ) ;
#15903=CARTESIAN_POINT ( 'NONE',  ( 0.000000000000000000, 0.000000000000000000, 0.000000000000000000 ) ) ;
#15958=VERTEX_POINT ( 'NONE', #2409 ) ;
#15977=ORIENTED_EDGE ( 'NONE', *, *, #14886, .F. ) ;
#15978=CARTESIAN_POINT ( 'NONE',  ( 209.9044635914013668, 29.65591986667770641, -11.50010063814821315 ) ) ;
#16037=EDGE_CURVE ( 'NONE', #15664, #4012, #1579, .T. ) ;
#16043=CARTESIAN_POINT ( 'NONE',  ( 209.2413142193426268, 30.98740296050068821, -15.88417608133634751 ) ) ;
#16081=CARTESIAN_POINT ( 'NONE',  ( 211.3675436807652375, 27.51476459780207406, -13.34822117963639698 ) ) ;
#16091=EDGE_CURVE ( 'NONE', #7353, #19322, #12378, .T. ) ;
#16106=EDGE_CURVE ( 'NONE', #17685, #4227, #7481, .T. ) ;
#16115=VECTOR ( 'NONE', #13587, 1000.000000000000227 ) ;
#16121=CARTESIAN_POINT ( 'NONE',  ( 201.8234976231972553, 26.52995303002162331, -14.00000000000004619 ) ) ;
#16140=CARTESIAN_POINT ( 'NONE',  ( 209.9065677398659204, 29.65222043997809109, -16.50006186076872083 ) ) ;
#16147=DIRECTION ( 'NONE',  ( 7.930164461608273850E-15, 3.965082230804136925E-15, -1.000000000000000000 ) ) ;
#16181=CARTESIAN_POINT ( 'NONE',  ( 209.4060512283256230, 30.62413204007591716, -11.83134160488075715 ) ) ;
#16225=DIRECTION ( 'NONE',  ( 0.5000000000000044409, -0.8660254037844360431, -4.006172263299080068E-16 ) ) ;
#16267=ADVANCED_FACE ( 'NONE', ( #14497 ), #19251, .T. ) ;
#16272=CARTESIAN_POINT ( 'NONE',  ( 210.8927598318763899, 28.12706523984405038, -12.11611233826046963 ) ) ;
#16318=CARTESIAN_POINT ( 'NONE',  ( 190.9712048706970506, 36.57158503910383729, -18.97089895516968028 ) ) ;
#16364=CARTESIAN_POINT ( 'NONE',  ( 190.7433706042750146, 35.72129598111152404, -9.000000000000062172 ) ) ;
#16371=LINE ( 'NONE', #3734, #942 ) ;
#16377=ORIENTED_EDGE ( 'NONE', *, *, #6874, .F. ) ;
#16397=DIRECTION ( 'NONE',  ( 0.000000000000000000, -1.000000000000000000, -3.469446951953589044E-16 ) ) ;
#16420=DIRECTION ( 'NONE',  ( 0.5000000000000057732, -0.8660254037844353769, 0.000000000000000000 ) ) ;
#16425=CARTESIAN_POINT ( 'NONE',  ( 157.3972143829815309, 45.33639716978957068, -22.00000000000007816 ) ) ;
#16433=CARTESIAN_POINT ( 'NONE',  ( 186.7423748293213066, 36.79335956793068618, -19.00000000000003908 ) ) ;
#16447=CARTESIAN_POINT ( 'NONE',  ( 191.0833833835253301, 36.99024094849632860, -9.087049258353282255 ) ) ;
#16516=EDGE_CURVE ( 'NONE', #270, #12839, #7599, .T. ) ;
#16518=FACE_OUTER_BOUND ( 'NONE', #9511, .T. ) ;
#16519=EDGE_CURVE ( 'NONE', #16924, #17685, #19809, .T. ) ;
#16535=AXIS2_PLACEMENT_3D ( 'NONE', #2578, #13916, #14029 ) ;
#16561=EDGE_CURVE ( 'NONE', #15958, #270, #13361, .T. ) ;
#16562=ORIENTED_EDGE ( 'NONE', *, *, #8821, .F. ) ;
#16595=CARTESIAN_POINT ( 'NONE',  ( 201.9876788769632299, 25.95811253888945203, -15.19853025469339869 ) ) ;
#16623=DIRECTION ( 'NONE',  ( -0.5000000000000044409, 0.8660254037844360431, 4.006172263299080068E-16 ) ) ;
#16694=ORIENTED_EDGE ( 'NONE', *, *, #16091, .T. ) ;
#16716=ORIENTED_EDGE ( 'NONE', *, *, #8472, .F. ) ;
#16720=ORIENTED_EDGE ( 'NONE', *, *, #5295, .F. ) ;
#16791=DIRECTION ( 'NONE',  ( 0.000000000000000000, 8.673617379884020681E-16, -1.000000000000000000 ) ) ;
#16816=CARTESIAN_POINT ( 'NONE',  ( 194.7177224586705222, 20.69538101841223821, -14.00000000000005329 ) ) ;
#16854=CARTESIAN_POINT ( 'NONE',  ( 157.3972143829815309, 45.33639716978955647, -6.000000000000052403 ) ) ;
#16894=EDGE_CURVE ( 'NONE', #17359, #19103, #7923, .T. ) ;
#16912=CARTESIAN_POINT ( 'NONE',  ( 202.8024860698635337, 24.48684974555284910, -15.30893474520620501 ) ) ;
#16924=VERTEX_POINT ( 'NONE', #9297 ) ;
#16945=CARTESIAN_POINT ( 'NONE',  ( 203.3160137783235371, 23.93889567138195673, -13.80219421229064736 ) ) ;
#16985=CARTESIAN_POINT ( 'NONE',  ( 191.5478494775925640, 36.18576207517880050, -14.00000000000006395 ) ) ;
#17005=CARTESIAN_POINT ( 'NONE',  ( 172.3972143829817014, 19.35563505625649583, -14.00000000000007461 ) ) ;
#17028=CARTESIAN_POINT ( 'NONE',  ( 215.1183575532813848, 35.36044452787341896, -14.00000000000004441 ) ) ;
#17044=CARTESIAN_POINT ( 'NONE',  ( 183.9132435853528307, 37.55142300003367950, -14.00000000000003730 ) ) ;
#17082=FACE_OUTER_BOUND ( 'NONE', #2091, .T. ) ;
#17085=EDGE_CURVE ( 'NONE', #19103, #4227, #14532, .T. ) ;
#17088=VERTEX_POINT ( 'NONE', #4957 ) ;
#17113=ORIENTED_EDGE ( 'NONE', *, *, #11750, .T. ) ;
#17178=DIRECTION ( 'NONE',  ( 0.5000000000000044409, -0.8660254037844360431, 0.000000000000000000 ) ) ;
#17182=DIRECTION ( 'NONE',  ( -0.8660254037844360431, -0.5000000000000045519, 0.000000000000000000 ) ) ;
#17224=CARTESIAN_POINT ( 'NONE',  ( 177.1791022559528983, 56.75747545832872731, 0.9999999999999431566 ) ) ;
#17259=DIRECTION ( 'NONE',  ( 0.5000000000000044409, -0.8660254037844360431, 0.000000000000000000 ) ) ;
#17322=ORIENTED_EDGE ( 'NONE', *, *, #4715, .T. ) ;
#17323=DIRECTION ( 'NONE',  ( 0.000000000000000000, -1.000000000000000000, -4.616915249250367527E-16 ) ) ;
#17355=DIRECTION ( 'NONE',  ( -0.8660254037844344888, -0.5000000000000069944, 0.000000000000000000 ) ) ;
#17359=VERTEX_POINT ( 'NONE', #13001 ) ;
#17390=PLANE ( 'NONE',  #8905 ) ;
#17409=CARTESIAN_POINT ( 'NONE',  ( 211.2092941256368306, 27.71181611822996160, -15.25318819445429597 ) ) ;
#17482=CIRCLE ( 'NONE', #18485, 5.000000000000002665 ) ;
#17512=CARTESIAN_POINT ( 'NONE',  ( 178.2433706042749009, 57.37193107572242923, -14.00000000000002842 ) ) ;
#17528=DIRECTION ( 'NONE',  ( 0.5000000000000045519, -0.8660254037844360431, -4.006172263299080561E-16 ) ) ;
#17536=DIRECTION ( 'NONE',  ( 0.5000000000000057732, -0.8660254037844353769, 0.000000000000000000 ) ) ;
#17567=AXIS2_PLACEMENT_3D ( 'NONE', #13621, #15332, #14044 ) ;
#17577=DIRECTION ( 'NONE',  ( 0.8660254037844354880, 0.5000000000000053291, 0.000000000000000000 ) ) ;
#17578=DIRECTION ( 'NONE',  ( -0.8660254037844361541, -0.5000000000000045519, -4.336808689942050770E-16 ) ) ;
#17587=EDGE_LOOP ( 'NONE', ( #11131, #11687, #1236, #9512, #502, #7502 ) ) ;
#17634=CIRCLE ( 'NONE', #4100, 5.000000000000002665 ) ;
#17640=UNCERTAINTY_MEASURE_WITH_UNIT (LENGTH_MEASURE( 1.000000000000000082E-05 ), #13415, 'distance_accuracy_value', 'NONE');
#17662=DIRECTION ( 'NONE',  ( -0.8660254037844360431, -0.5000000000000045519, -4.336808689942050277E-16 ) ) ;
#17685=VERTEX_POINT ( 'NONE', #7010 ) ;
#17712=ORIENTED_EDGE ( 'NONE', *, *, #20067, .T. ) ;
#17729=CARTESIAN_POINT ( 'NONE',  ( 210.8238100345766384, 28.21933447757778168, -15.99832059698782061 ) ) ;
#17735=DIRECTION ( 'NONE',  ( 0.5000000000000044409, -0.8660254037844360431, 0.000000000000000000 ) ) ;
#17776=EDGE_CURVE ( 'NONE', #3226, #13023, #15531, .T. ) ;
#17785=ORIENTED_EDGE ( 'NONE', *, *, #5886, .F. ) ;
#17818=DIRECTION ( 'NONE',  ( -7.930164461608272272E-15, -3.965082230804136136E-15, -1.000000000000000000 ) ) ;
#17826=CARTESIAN_POINT ( 'NONE',  ( 211.4089789608015622, 27.46411792184940026, -14.32816039117628115 ) ) ;
#17868=VECTOR ( 'NONE', #13847, 1000.000000000000114 ) ;
#17873=CARTESIAN_POINT ( 'NONE',  ( 209.1090394831926176, 31.29886781828238895, -12.47428928897383749 ) ) ;
#17882=VECTOR ( 'NONE', #19847, 1000.000000000000114 ) ;
#17936=ADVANCED_FACE ( 'NONE', ( #8833 ), #7551, .F. ) ;
#17948=VERTEX_POINT ( 'NONE', #17005 ) ;
#17957=CARTESIAN_POINT ( 'NONE',  ( 188.9132435853528591, 28.89116896218935082, -14.00000000000004086 ) ) ;
#17969=EDGE_CURVE ( 'NONE', #4227, #19623, #15539, .T. ) ;
#17977=DIRECTION ( 'NONE',  ( -0.8660254037844360431, -0.5000000000000045519, -4.336808689942050277E-16 ) ) ;
#17999=CARTESIAN_POINT ( 'NONE',  ( 169.8972143829816730, 23.68576207517868326, -14.00000000000007461 ) ) ;
#18016=PLANE ( 'NONE',  #7453 ) ;
#18044=CARTESIAN_POINT ( 'NONE',  ( 177.1791022559528983, 56.75747545832872731, 0.9999999999999431566 ) ) ;
#18045=CARTESIAN_POINT ( 'NONE',  ( 190.7433706042750146, 35.72129598111152404, -9.000000000000062172 ) ) ;
#18066=AXIS2_PLACEMENT_3D ( 'NONE', #4777, #9642, #1500 ) ;
#18073=CARTESIAN_POINT ( 'NONE',  ( 209.0398851729401315, 31.46936297222353929, -12.74687664482581795 ) ) ;
#18097=AXIS2_PLACEMENT_3D ( 'NONE', #586, #19862, #18281 ) ;
#18125=ORIENTED_EDGE ( 'NONE', *, *, #16894, .F. ) ;
#18132=DIRECTION ( 'NONE',  ( -0.8660254037844361541, -0.5000000000000044409, 0.000000000000000000 ) ) ;
#18143=CARTESIAN_POINT ( 'NONE',  ( 202.9102931164051711, 24.36002564953663097, -12.80119896869108764 ) ) ;
#18205=ORIENTED_EDGE ( 'NONE', *, *, #17776, .F. ) ;
#18212=CARTESIAN_POINT ( 'NONE',  ( 179.0478494775924503, 57.83639716978969147, -18.91295074164678169 ) ) ;
#18229=VECTOR ( 'NONE', #16791, 1000.000000000000000 ) ;
#18232=EDGE_LOOP ( 'NONE', ( #4973, #9218, #14392, #11983 ) ) ;
#18233=AXIS2_PLACEMENT_3D ( 'NONE', #15903, #1274, #19656 ) ;
#18238=ADVANCED_FACE ( 'NONE', ( #7425 ), #20576, .F. ) ;
#18261=CARTESIAN_POINT ( 'NONE',  ( 159.9952905943348469, 46.83639716978958489, -29.00000000000006750 ) ) ;
#18281=DIRECTION ( 'NONE',  ( 0.5000000000000057732, -0.8660254037844353769, 0.000000000000000000 ) ) ;
#18289=CARTESIAN_POINT ( 'NONE',  ( 202.3246710188176110, 25.20128250578996187, -15.50000755803645802 ) ) ;
#18294=CYLINDRICAL_SURFACE ( 'NONE', #5395, 1.499999999999990896 ) ;
#18333=VERTEX_POINT ( 'NONE', #1403 ) ;
#18364=ORIENTED_EDGE ( 'NONE', *, *, #17969, .T. ) ;
#18417=CIRCLE ( 'NONE', #9253, 4.999999999999978684 ) ;
#18445=DIRECTION ( 'NONE',  ( 0.000000000000000000, 8.673617379884020681E-16, -1.000000000000000000 ) ) ;
#18474=DIRECTION ( 'NONE',  ( 0.5000000000000044409, -0.8660254037844360431, -4.006172263299080068E-16 ) ) ;
#18485=AXIS2_PLACEMENT_3D ( 'NONE', #6708, #17977, #6606 ) ;
#18509=CARTESIAN_POINT ( 'NONE',  ( 201.8425266500695727, 26.45120969970218283, -14.48650656672420389 ) ) ;
#18517=DIRECTION ( 'NONE',  ( 0.8660254037844355990, 0.5000000000000051070, -1.748523119690306661E-16 ) ) ;
#18519=DIRECTION ( 'NONE',  ( -0.8660254037844360431, -0.5000000000000045519, -4.336808689942050277E-16 ) ) ;
#18564=CARTESIAN_POINT ( 'NONE',  ( 177.1791022559528983, 56.75747545832872731, -14.00000000000006395 ) ) ;
#18596=CARTESIAN_POINT ( 'NONE',  ( 198.9132435853529728, 11.57066088650059932, -14.00000000000004974 ) ) ;
#18607=CARTESIAN_POINT ( 'NONE',  ( 202.4235407509943911, 25.03004461941911529, -15.49999243318709574 ) ) ;
#18776=DIRECTION ( 'NONE',  ( -0.8660254037844360431, -0.5000000000000045519, 0.000000000000000000 ) ) ;
#18825=DIRECTION ( 'NONE',  ( -1.000000000000000000, 0.000000000000000000, 3.517351572405780687E-16 ) ) ;
#18850=ORIENTED_EDGE ( 'NONE', *, *, #8879, .T. ) ;
#18884=EDGE_CURVE ( 'NONE', #12839, #14228, #299, .T. ) ;
#18892=EDGE_CURVE ( 'NONE', #2720, #9060, #14546, .T. ) ;
#18966=VECTOR ( 'NONE', #3983, 1000.000000000000114 ) ;
#19009=PLANE ( 'NONE',  #20012 ) ;
#19015=ADVANCED_FACE ( 'NONE', ( #16518 ), #8446, .T. ) ;
#19045=STYLED_ITEM('',(#20974),#10635);
#19051=DIRECTION ( 'NONE',  ( 0.5000000000000044409, -0.8660254037844360431, -4.006172263299080068E-16 ) ) ;
#19086=AXIS2_PLACEMENT_3D ( 'NONE', #12444, #14036, #2893 ) ;
#19095=ORIENTED_EDGE ( 'NONE', *, *, #17085, .F. ) ;
#19103=VERTEX_POINT ( 'NONE', #10345 ) ;
#19128=FACE_OUTER_BOUND ( 'NONE', #6499, .T. ) ;
#19168=ORIENTED_EDGE ( 'NONE', *, *, #8821, .T. ) ;
#19174=VECTOR ( 'NONE', #19051, 1000.000000000000114 ) ;
#19249=CARTESIAN_POINT ( 'NONE',  ( 211.4089818235499365, 27.46411299765594904, -13.67111640670284167 ) ) ;
#19251=PLANE ( 'NONE',  #5285 ) ;
#19260=( LENGTH_UNIT ( ) NAMED_UNIT ( * ) SI_UNIT ( .MILLI., .METRE. ) );
#19263=PRODUCT_DEFINITION_FORMATION_WITH_SPECIFIED_SOURCE ( 'ANY', '', #783, .NOT_KNOWN. ) ;
#19273=ORIENTED_EDGE ( 'NONE', *, *, #14886, .T. ) ;
#19305=CARTESIAN_POINT ( 'NONE',  ( 208.9252846479952836, 31.76596812687403926, -14.32921182609460864 ) ) ;
#19318=DIRECTION ( 'NONE',  ( -0.8660254037844361541, -0.5000000000000042188, 0.000000000000000000 ) ) ;
#19321=ORIENTED_EDGE ( 'NONE', *, *, #18884, .T. ) ;
#19322=VERTEX_POINT ( 'NONE', #8637 ) ;
#19327=DIRECTION ( 'NONE',  ( -0.8660254037844360431, -0.5000000000000045519, -4.336808689942049784E-16 ) ) ;
#19407=CARTESIAN_POINT ( 'NONE',  ( 211.0319935650719572, 27.94071137980556685, -15.65309054528693089 ) ) ;
#19429=ADVANCED_FACE ( 'NONE', ( #13524 ), #11938, .F. ) ;
#19530=CARTESIAN_POINT ( 'NONE',  ( 167.3972143829816446, 28.01588909410086004, -14.00000000000007461 ) ) ;
#19605=CYLINDRICAL_SURFACE ( 'NONE', #6178, 5.000000000000002665 ) ;
#19623=VERTEX_POINT ( 'NONE', #20785 ) ;
#19629=ORIENTED_EDGE ( 'NONE', *, *, #18892, .T. ) ;
#19656=DIRECTION ( 'NONE',  ( 1.000000000000000000, 0.000000000000000000, 0.000000000000000000 ) ) ;
#19722=CARTESIAN_POINT ( 'NONE',  ( 201.8619877917642782, 26.37553173410844565, -13.33277734556806138 ) ) ;
#19751=EDGE_CURVE ( 'NONE', #17088, #9882, #14980, .T. ) ;
#19807=VECTOR ( 'NONE', #6770, 1000.000000000000000 ) ;
#19809=LINE ( 'NONE', #120, #13445 ) ;
#19827=CARTESIAN_POINT ( 'NONE',  ( 202.0446258486138902, 25.79888835193206376, -12.69000053959321939 ) ) ;
#19847=DIRECTION ( 'NONE',  ( 0.8660254037844360431, 0.5000000000000044409, 4.336808689942049290E-16 ) ) ;
#19862=DIRECTION ( 'NONE',  ( -0.8660254037844360431, -0.5000000000000045519, -4.336808689942049784E-16 ) ) ;
#19875=FACE_OUTER_BOUND ( 'NONE', #14322, .T. ) ;
#19921=CARTESIAN_POINT ( 'NONE',  ( 159.9952905943348469, 46.83639716978957068, 0.9999999999999386047 ) ) ;
#19978=CARTESIAN_POINT ( 'NONE',  ( 203.0966297564995671, 24.15688938925481111, -14.91618358615997408 ) ) ;
#20005=ORIENTED_EDGE ( 'NONE', *, *, #7003, .F. ) ;
#20012=AXIS2_PLACEMENT_3D ( 'NONE', #10725, #1512, #1305 ) ;
#20020=ORIENTED_EDGE ( 'NONE', *, *, #18892, .F. ) ;
#20022=ORIENTED_EDGE ( 'NONE', *, *, #20067, .F. ) ;
#20050=EDGE_CURVE ( 'NONE', #9060, #2720, #7464, .T. ) ;
#20067=EDGE_CURVE ( 'NONE', #10601, #12839, #2476, .T. ) ;
#20089=AXIS2_PLACEMENT_3D ( 'NONE', #5138, #11626, #16397 ) ;
#20091=CARTESIAN_POINT ( 'NONE',  ( 202.9101512355597094, 24.36019071069245356, -15.19895601951926878 ) ) ;
#20101=DIRECTION ( 'NONE',  ( 0.5000000000000015543, -0.8660254037844377084, 0.000000000000000000 ) ) ;
#20171=CARTESIAN_POINT ( 'NONE',  ( 177.1791022559528983, 56.75747545832872731, -14.00000000000006395 ) ) ;
#20186=( NAMED_UNIT ( * ) SI_UNIT ( $, .STERADIAN. ) SOLID_ANGLE_UNIT ( ) );
#20214=CARTESIAN_POINT ( 'NONE',  ( 182.5734976231970563, 59.87193107572243633, -14.00000000000002842 ) ) ;
#20228=LINE ( 'NONE', #5807, #2924 ) ;
#20249=ORIENTED_EDGE ( 'NONE', *, *, #665, .F. ) ;
#20291=AXIS2_PLACEMENT_3D ( 'NONE', #2632, #10660, #2733 ) ;
#20328=CARTESIAN_POINT ( 'NONE',  ( 201.9232776496033637, 26.15921614160104980, -13.00767012778560705 ) ) ;
#20363=VECTOR ( 'NONE', #10196, 1000.000000000000114 ) ;
#20370=DIRECTION ( 'NONE',  ( 0.5000000000000057732, -0.8660254037844353769, 0.000000000000000000 ) ) ;
#20375=VECTOR ( 'NONE', #15852, 1000.000000000000114 ) ;
#20392=EDGE_CURVE ( 'NONE', #14976, #16924, #16371, .T. ) ;
#20404=LINE ( 'NONE', #7781, #10495 ) ;
#20417=CARTESIAN_POINT ( 'NONE',  ( 190.1694833127194499, 64.25747545832879837, -14.00000000000006395 ) ) ;
#20436=EDGE_CURVE ( 'NONE', #10831, #784, #10192, .T. ) ;
#20457=FACE_OUTER_BOUND ( 'NONE', #4340, .T. ) ;
#20546=CARTESIAN_POINT ( 'NONE',  ( 159.9952905943347901, 46.83639716978954226, -6.000000000000052403 ) ) ;
#20576=CYLINDRICAL_SURFACE ( 'NONE', #297, 5.000000000000002665 ) ;
#20580=PLANE ( 'NONE',  #19086 ) ;
#20581=CARTESIAN_POINT ( 'NONE',  ( 191.1694443951678295, 35.60712985292573052, -9.000000000000063949 ) ) ;
#20682=CARTESIAN_POINT ( 'NONE',  ( 210.3241885033056917, 28.95566150434252961, -16.41972909894644417 ) ) ;
#20702=APPLICATION_CONTEXT ( 'automotive_design' ) ;
#20777=SHAPE_DEFINITION_REPRESENTATION ( #2657, #9638 ) ;
#20780=EDGE_LOOP ( 'NONE', ( #12860, #12810 ) ) ;
#20785=CARTESIAN_POINT ( 'NONE',  ( 182.3972143829817867, 2.035126980567763866, -22.00000000000009948 ) ) ;
#20786=DIRECTION ( 'NONE',  ( -0.8660254037844360431, -0.5000000000000044409, -4.336808689942049290E-16 ) ) ;
#20787=EDGE_CURVE ( 'NONE', #19103, #17088, #750, .T. ) ;
#20822=CARTESIAN_POINT ( 'NONE',  ( 208.9194833127196489, 31.78152281641241572, -14.00000000000007816 ) ) ;
#20842=( BOUNDED_CURVE ( )  B_SPLINE_CURVE ( 3, ( #5118, #1642, #154, #11602 ),
 .UNSPECIFIED., .F., .F. ) 
 B_SPLINE_CURVE_WITH_KNOTS ( ( 4, 4 ),
 ( 1.404087049333884217E-16, 1.570796326794897002 ),
 .UNSPECIFIED. ) 
 CURVE ( )  GEOMETRIC_REPRESENTATION_ITEM ( )  RATIONAL_B_SPLINE_CURVE ( ( 1.000000000000000000, 0.8047378541243649375, 0.8047378541243649375, 1.000000000000000000 ) ) 
 REPRESENTATION_ITEM ( '' )  );
#20883=EDGE_CURVE ( 'NONE', #14976, #17359, #849, .T. ) ;
#20902=CYLINDRICAL_SURFACE ( 'NONE', #13771, 5.000000000000002665 ) ;
#20909=CARTESIAN_POINT ( 'NONE',  ( 189.6713070174558311, 31.72030020615783386, -19.00000000000004263 ) ) ;
#20913=ORIENTED_EDGE ( 'NONE', *, *, #1267, .F. ) ;
#20921=CARTESIAN_POINT ( 'NONE',  ( 210.0696016554955463, 29.36982461651845711, -11.49990028153587218 ) ) ;
#20968=COLOUR_RGB('Light Blue',0.38,0.62,0.78);
#20969=FILL_AREA_STYLE_COLOUR('',#20968);
#20970=FILL_AREA_STYLE('',(#20969));
#20971=SURFACE_STYLE_FILL_AREA(#20970);
#20972=SURFACE_SIDE_STYLE('',(#20971));
#20973=SURFACE_STYLE_USAGE(.BOTH.,#20972);
#20974=PRESENTATION_STYLE_ASSIGNMENT((#20973));
ENDSEC;
END-ISO-10303-21;
